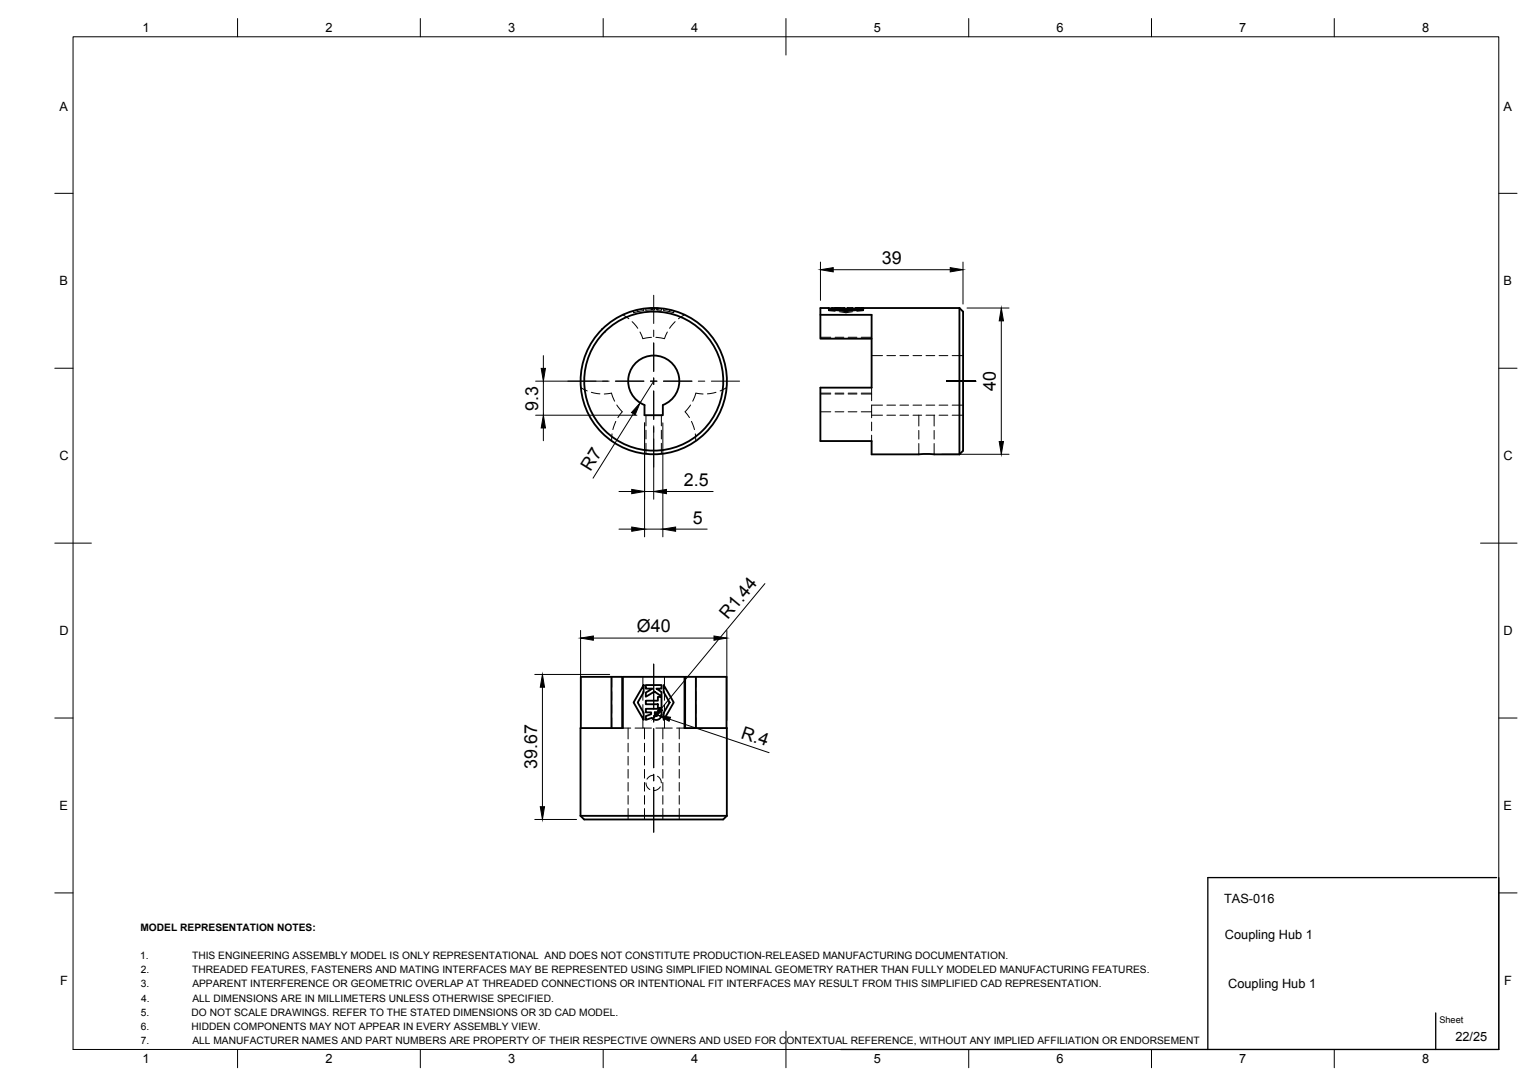
ISO-10303-21;
HEADER;
/* Generated by software containing ST-Developer
 * from STEP Tools, Inc. (www.steptools.com) 
 */

FILE_DESCRIPTION(
/* description */ ('STEP AP214'),
/* implementation_level */ '2;1');

FILE_NAME(
/* name */ 'Coupling Hub 1.step',
/* time_stamp */ '2026-11-15T14:55:55-08:00',
/* author */ (''),
/* organization */ (''),
/* preprocessor_version */ 'ST-DEVELOPER v20.2',
/* originating_system */ 'Autodesk Translation Framework v15.17.0.0',
/* authorisation */ '');

FILE_SCHEMA (('AUTOMOTIVE_DESIGN { 1 0 10303 214 3 1 1 }'));
ENDSEC;

DATA;
#10=MECHANICAL_DESIGN_GEOMETRIC_PRESENTATION_REPRESENTATION('',(#941),#57079);
#66=ELLIPSE('',#25719,40.0000000130718,20.0000000134373);
#67=ELLIPSE('',#25720,39.9999999264935,19.999999930827);
#68=ELLIPSE('',#25721,39.9999999974836,19.9999999977429);
#69=ELLIPSE('',#25722,40.0000000047116,20.0000000045204);
#70=ELLIPSE('',#25723,23.3867968076182,20.);
#71=ELLIPSE('',#25724,23.386796807644,20.);
#72=ELLIPSE('',#25728,24.1243589702644,20.);
#73=ELLIPSE('',#25729,24.124358970134,20.);
#74=ELLIPSE('',#25730,39.999999976902,19.9999999789991);
#75=ELLIPSE('',#25731,40.0000000049323,20.0000000047275);
#76=ELLIPSE('',#25732,39.9999999975502,19.999999997805);
#77=ELLIPSE('',#25733,39.9999999389236,19.9999999427079);
#78=ELLIPSE('',#25748,22.8021268874529,19.5);
#79=ELLIPSE('',#25751,22.8021268874277,19.5);
#80=ELLIPSE('',#25754,23.5212499960078,19.5);
#81=ELLIPSE('',#25764,23.5212499958807,19.5);
#82=ELLIPSE('',#25767,39.0000000024375,19.500000002367);
#83=ELLIPSE('',#25768,39.0000000667235,19.500000064201);
#84=ELLIPSE('',#25769,38.9999999995571,19.5000000004649);
#85=ELLIPSE('',#25770,38.999999996593,19.4999999968888);
#86=ELLIPSE('',#25779,38.9999999955418,19.4999999959037);
#87=ELLIPSE('',#25781,38.999999997527,19.4999999977637);
#88=ELLIPSE('',#25784,39.0000000253793,19.5000000249782);
#89=ELLIPSE('',#25786,39.0000000418424,19.5000000405918);
#844=B_SPLINE_CURVE_WITH_KNOTS('',3,(#51735,#51736,#51737,#51738,#51739,
#51740,#51741,#51742,#51743,#51744,#51745,#51746,#51747,#51748,#51749,#51750,
#51751,#51752),.UNSPECIFIED.,.F.,.F.,(4,2,2,2,2,2,2,2,4),(0.,0.0151925643701926,
0.0303851287403852,0.045584296496648,0.0607834642529108,0.0759910091953897,
0.0911985541378687,0.106391953286869,0.121585352435869),.UNSPECIFIED.);
#845=B_SPLINE_CURVE_WITH_KNOTS('',3,(#51844,#51845,#51846,#51847,#51848,
#51849,#51850,#51851,#51852,#51853,#51854,#51855,#51856,#51857,#51858,#51859,
#51860,#51861),.UNSPECIFIED.,.F.,.F.,(4,2,2,2,2,2,2,2,4),(0.316667444606564,
0.395834141831916,0.475000839057267,0.554167864135198,0.633334889213128,
0.712501914291059,0.791668939368989,0.870835636594341,0.950002333819692),
 .UNSPECIFIED.);
#846=B_SPLINE_CURVE_WITH_KNOTS('',3,(#51863,#51864,#51865,#51866,#51867,
#51868,#51869,#51870,#51871,#51872),.UNSPECIFIED.,.F.,.F.,(4,2,2,2,4),(-1.26666977842626,
-1.18750275334833,-1.10833572827039,-1.02916903104504,-0.950002333819692),
 .UNSPECIFIED.);
#847=B_SPLINE_CURVE_WITH_KNOTS('',3,(#51873,#51874,#51875,#51876,#51877,
#51878,#51879,#51880,#51881,#51882),.UNSPECIFIED.,.F.,.F.,(4,2,2,2,4),(0.950002333819692,
1.02916903104504,1.1083357282704,1.18750275334833,1.26666977842626),
 .UNSPECIFIED.);
#848=B_SPLINE_CURVE_WITH_KNOTS('',3,(#51888,#51889,#51890,#51891,#51892,
#51893,#51894,#51895,#51896,#51897,#51898,#51899,#51900,#51901,#51902,#51903),
 .UNSPECIFIED.,.F.,.F.,(4,2,2,2,2,2,2,4),(-0.779979052988675,-0.757912790448093,
-0.703814302563526,-0.64971581467896,-0.595510917659987,-0.541306020641014,
-0.487185868025911,-0.433065715410808),.UNSPECIFIED.);
#849=B_SPLINE_CURVE_WITH_KNOTS('',3,(#52126,#52127,#52128,#52129,#52130,
#52131,#52132,#52133,#52134,#52135,#52136,#52137,#52138,#52139,#52140,#52141),
 .UNSPECIFIED.,.F.,.F.,(4,2,2,2,2,2,2,4),(0.43308109743951,0.487202501340474,
0.541323905241438,0.595534461493003,0.649745017744569,0.703843614398011,
0.757942211051454,0.780009479202147),.UNSPECIFIED.);
#850=B_SPLINE_CURVE_WITH_KNOTS('',3,(#52173,#52174,#52175,#52176,#52177,
#52178,#52179,#52180,#52181,#52182,#52183,#52184,#52185,#52186,#52187,#52188,
#52189,#52190),.UNSPECIFIED.,.F.,.F.,(4,2,2,2,2,2,2,2,4),(0.121587491028333,
0.136780909575281,0.151974328122229,0.167182628159423,0.182390928196617,
0.197590414964019,0.212789901731421,0.227982441894043,0.243174982056666),
 .UNSPECIFIED.);
#881=SHAPE_REPRESENTATION_RELATIONSHIP('SRR','None',#57269,#910);
#910=ADVANCED_BREP_SHAPE_REPRESENTATION('',(#978),#57061);
#941=STYLED_ITEM('',(#57444),#978);
#978=MANIFOLD_SOLID_BREP('Body1',#24541);
#1139=FACE_BOUND('',#4148,.T.);
#1140=FACE_BOUND('',#4160,.T.);
#1141=FACE_BOUND('',#4166,.T.);
#1142=FACE_BOUND('',#4171,.T.);
#1143=FACE_BOUND('',#4172,.T.);
#1144=FACE_BOUND('',#4173,.T.);
#1145=FACE_BOUND('',#4174,.T.);
#1146=FACE_BOUND('',#4175,.T.);
#1147=FACE_BOUND('',#4225,.T.);
#1550=PLANE('',#25658);
#1551=PLANE('',#25663);
#1552=PLANE('',#25670);
#1553=PLANE('',#25675);
#1554=PLANE('',#25692);
#1555=PLANE('',#25705);
#1556=PLANE('',#25707);
#1557=PLANE('',#25708);
#1558=PLANE('',#25739);
#1559=PLANE('',#25740);
#1560=PLANE('',#25741);
#1561=PLANE('',#25742);
#1562=PLANE('',#25743);
#1563=PLANE('',#25744);
#1564=PLANE('',#25745);
#1565=PLANE('',#25746);
#1566=PLANE('',#25747);
#1567=PLANE('',#25749);
#1568=PLANE('',#25750);
#1569=PLANE('',#25752);
#1570=PLANE('',#25753);
#1571=PLANE('',#25755);
#1572=PLANE('',#25757);
#1573=PLANE('',#25758);
#1574=PLANE('',#25760);
#1575=PLANE('',#25761);
#1576=PLANE('',#25763);
#1577=PLANE('',#25771);
#1578=PLANE('',#25772);
#1579=PLANE('',#25773);
#1580=PLANE('',#25774);
#1581=PLANE('',#25775);
#1582=PLANE('',#25776);
#1583=PLANE('',#25777);
#1584=PLANE('',#25778);
#1585=PLANE('',#25780);
#1586=PLANE('',#25782);
#1587=PLANE('',#25783);
#1588=PLANE('',#25785);
#1589=PLANE('',#25788);
#1590=PLANE('',#25790);
#1591=PLANE('',#25791);
#1592=PLANE('',#25794);
#1593=PLANE('',#25795);
#1594=PLANE('',#25797);
#1595=PLANE('',#25798);
#1596=PLANE('',#25800);
#1597=PLANE('',#25801);
#1598=PLANE('',#25803);
#1599=PLANE('',#25805);
#2122=CONICAL_SURFACE('',#25666,19.5,0.785398163397448);
#2632=FACE_OUTER_BOUND('',#4146,.T.);
#2633=FACE_OUTER_BOUND('',#4147,.T.);
#2634=FACE_OUTER_BOUND('',#4149,.T.);
#2635=FACE_OUTER_BOUND('',#4150,.T.);
#2636=FACE_OUTER_BOUND('',#4151,.T.);
#2637=FACE_OUTER_BOUND('',#4152,.T.);
#2638=FACE_OUTER_BOUND('',#4153,.T.);
#2639=FACE_OUTER_BOUND('',#4154,.T.);
#2640=FACE_OUTER_BOUND('',#4155,.T.);
#2641=FACE_OUTER_BOUND('',#4156,.T.);
#2642=FACE_OUTER_BOUND('',#4157,.T.);
#2643=FACE_OUTER_BOUND('',#4158,.T.);
#2644=FACE_OUTER_BOUND('',#4159,.T.);
#2645=FACE_OUTER_BOUND('',#4161,.T.);
#2646=FACE_OUTER_BOUND('',#4162,.T.);
#2647=FACE_OUTER_BOUND('',#4163,.T.);
#2648=FACE_OUTER_BOUND('',#4164,.T.);
#2649=FACE_OUTER_BOUND('',#4165,.T.);
#2650=FACE_OUTER_BOUND('',#4167,.T.);
#2651=FACE_OUTER_BOUND('',#4168,.T.);
#2652=FACE_OUTER_BOUND('',#4169,.T.);
#2653=FACE_OUTER_BOUND('',#4170,.T.);
#2654=FACE_OUTER_BOUND('',#4176,.T.);
#2655=FACE_OUTER_BOUND('',#4177,.T.);
#2656=FACE_OUTER_BOUND('',#4178,.T.);
#2657=FACE_OUTER_BOUND('',#4179,.T.);
#2658=FACE_OUTER_BOUND('',#4180,.T.);
#2659=FACE_OUTER_BOUND('',#4181,.T.);
#2660=FACE_OUTER_BOUND('',#4182,.T.);
#2661=FACE_OUTER_BOUND('',#4183,.T.);
#2662=FACE_OUTER_BOUND('',#4184,.T.);
#2663=FACE_OUTER_BOUND('',#4185,.T.);
#2664=FACE_OUTER_BOUND('',#4186,.T.);
#2665=FACE_OUTER_BOUND('',#4187,.T.);
#2666=FACE_OUTER_BOUND('',#4188,.T.);
#2667=FACE_OUTER_BOUND('',#4189,.T.);
#2668=FACE_OUTER_BOUND('',#4190,.T.);
#2669=FACE_OUTER_BOUND('',#4191,.T.);
#2670=FACE_OUTER_BOUND('',#4192,.T.);
#2671=FACE_OUTER_BOUND('',#4193,.T.);
#2672=FACE_OUTER_BOUND('',#4194,.T.);
#2673=FACE_OUTER_BOUND('',#4195,.T.);
#2674=FACE_OUTER_BOUND('',#4196,.T.);
#2675=FACE_OUTER_BOUND('',#4197,.T.);
#2676=FACE_OUTER_BOUND('',#4198,.T.);
#2677=FACE_OUTER_BOUND('',#4199,.T.);
#2678=FACE_OUTER_BOUND('',#4200,.T.);
#2679=FACE_OUTER_BOUND('',#4201,.T.);
#2680=FACE_OUTER_BOUND('',#4202,.T.);
#2681=FACE_OUTER_BOUND('',#4203,.T.);
#2682=FACE_OUTER_BOUND('',#4204,.T.);
#2683=FACE_OUTER_BOUND('',#4205,.T.);
#2684=FACE_OUTER_BOUND('',#4206,.T.);
#2685=FACE_OUTER_BOUND('',#4207,.T.);
#2686=FACE_OUTER_BOUND('',#4208,.T.);
#2687=FACE_OUTER_BOUND('',#4209,.T.);
#2688=FACE_OUTER_BOUND('',#4210,.T.);
#2689=FACE_OUTER_BOUND('',#4211,.T.);
#2690=FACE_OUTER_BOUND('',#4212,.T.);
#2691=FACE_OUTER_BOUND('',#4213,.T.);
#2692=FACE_OUTER_BOUND('',#4214,.T.);
#2693=FACE_OUTER_BOUND('',#4215,.T.);
#2694=FACE_OUTER_BOUND('',#4216,.T.);
#2695=FACE_OUTER_BOUND('',#4217,.T.);
#2696=FACE_OUTER_BOUND('',#4218,.T.);
#2697=FACE_OUTER_BOUND('',#4219,.T.);
#2698=FACE_OUTER_BOUND('',#4220,.T.);
#2699=FACE_OUTER_BOUND('',#4221,.T.);
#2700=FACE_OUTER_BOUND('',#4222,.T.);
#2701=FACE_OUTER_BOUND('',#4223,.T.);
#2702=FACE_OUTER_BOUND('',#4224,.T.);
#4146=EDGE_LOOP('',(#18044,#18045,#18046,#18047));
#4147=EDGE_LOOP('',(#18048));
#4148=EDGE_LOOP('',(#18049,#18050,#18051,#18052));
#4149=EDGE_LOOP('',(#18053,#18054,#18055,#18056));
#4150=EDGE_LOOP('',(#18057,#18058,#18059,#18060));
#4151=EDGE_LOOP('',(#18061,#18062,#18063,#18064));
#4152=EDGE_LOOP('',(#18065,#18066,#18067,#18068));
#4153=EDGE_LOOP('',(#18069,#18070,#18071,#18072));
#4154=EDGE_LOOP('',(#18073,#18074,#18075,#18076));
#4155=EDGE_LOOP('',(#18077,#18078,#18079,#18080));
#4156=EDGE_LOOP('',(#18081,#18082,#18083,#18084));
#4157=EDGE_LOOP('',(#18085,#18086,#18087,#18088));
#4158=EDGE_LOOP('',(#18089,#18090,#18091,#18092));
#4159=EDGE_LOOP('',(#18093,#18094,#18095,#18096,#18097,#18098,#18099,#18100,
#18101,#18102,#18103,#18104,#18105));
#4160=EDGE_LOOP('',(#18106,#18107,#18108,#18109));
#4161=EDGE_LOOP('',(#18110,#18111,#18112,#18113));
#4162=EDGE_LOOP('',(#18114,#18115,#18116,#18117));
#4163=EDGE_LOOP('',(#18118,#18119,#18120,#18121));
#4164=EDGE_LOOP('',(#18122,#18123,#18124,#18125));
#4165=EDGE_LOOP('',(#18126,#18127,#18128,#18129));
#4166=EDGE_LOOP('',(#18130));
#4167=EDGE_LOOP('',(#18131,#18132,#18133,#18134));
#4168=EDGE_LOOP('',(#18135,#18136,#18137,#18138));
#4169=EDGE_LOOP('',(#18139,#18140,#18141,#18142,#18143,#18144));
#4170=EDGE_LOOP('',(#18145,#18146,#18147,#18148,#18149,#18150,#18151,#18152,
#18153,#18154,#18155,#18156,#18157,#18158,#18159,#18160,#18161,#18162,#18163,
#18164,#18165));
#4171=EDGE_LOOP('',(#18166,#18167,#18168,#18169,#18170,#18171,#18172,#18173,
#18174));
#4172=EDGE_LOOP('',(#18175,#18176,#18177,#18178,#18179,#18180,#18181,#18182));
#4173=EDGE_LOOP('',(#18183,#18184,#18185,#18186,#18187,#18188));
#4174=EDGE_LOOP('',(#18189,#18190,#18191,#18192,#18193,#18194,#18195,#18196,
#18197,#18198,#18199));
#4175=EDGE_LOOP('',(#18200,#18201,#18202,#18203,#18204,#18205));
#4176=EDGE_LOOP('',(#18206,#18207,#18208,#18209,#18210,#18211,#18212,#18213));
#4177=EDGE_LOOP('',(#18214,#18215,#18216,#18217));
#4178=EDGE_LOOP('',(#18218,#18219,#18220,#18221));
#4179=EDGE_LOOP('',(#18222,#18223,#18224,#18225));
#4180=EDGE_LOOP('',(#18226,#18227,#18228,#18229));
#4181=EDGE_LOOP('',(#18230,#18231,#18232,#18233));
#4182=EDGE_LOOP('',(#18234,#18235,#18236,#18237));
#4183=EDGE_LOOP('',(#18238,#18239,#18240,#18241));
#4184=EDGE_LOOP('',(#18242,#18243,#18244,#18245));
#4185=EDGE_LOOP('',(#18246,#18247,#18248,#18249));
#4186=EDGE_LOOP('',(#18250,#18251,#18252,#18253));
#4187=EDGE_LOOP('',(#18254,#18255,#18256,#18257));
#4188=EDGE_LOOP('',(#18258,#18259,#18260,#18261));
#4189=EDGE_LOOP('',(#18262,#18263,#18264,#18265));
#4190=EDGE_LOOP('',(#18266,#18267,#18268,#18269));
#4191=EDGE_LOOP('',(#18270,#18271,#18272,#18273));
#4192=EDGE_LOOP('',(#18274,#18275,#18276,#18277));
#4193=EDGE_LOOP('',(#18278,#18279,#18280,#18281));
#4194=EDGE_LOOP('',(#18282,#18283,#18284,#18285));
#4195=EDGE_LOOP('',(#18286,#18287,#18288,#18289));
#4196=EDGE_LOOP('',(#18290,#18291,#18292,#18293,#18294,#18295,#18296,#18297,
#18298,#18299,#18300));
#4197=EDGE_LOOP('',(#18301,#18302,#18303,#18304,#18305,#18306));
#4198=EDGE_LOOP('',(#18307,#18308,#18309,#18310));
#4199=EDGE_LOOP('',(#18311,#18312,#18313,#18314));
#4200=EDGE_LOOP('',(#18315,#18316,#18317,#18318));
#4201=EDGE_LOOP('',(#18319,#18320,#18321,#18322));
#4202=EDGE_LOOP('',(#18323,#18324,#18325,#18326));
#4203=EDGE_LOOP('',(#18327,#18328,#18329,#18330));
#4204=EDGE_LOOP('',(#18331,#18332,#18333,#18334));
#4205=EDGE_LOOP('',(#18335,#18336,#18337,#18338));
#4206=EDGE_LOOP('',(#18339,#18340,#18341,#18342));
#4207=EDGE_LOOP('',(#18343,#18344,#18345,#18346));
#4208=EDGE_LOOP('',(#18347,#18348,#18349,#18350));
#4209=EDGE_LOOP('',(#18351,#18352,#18353,#18354));
#4210=EDGE_LOOP('',(#18355,#18356,#18357,#18358,#18359,#18360));
#4211=EDGE_LOOP('',(#18361,#18362,#18363,#18364));
#4212=EDGE_LOOP('',(#18365,#18366,#18367,#18368));
#4213=EDGE_LOOP('',(#18369,#18370,#18371,#18372));
#4214=EDGE_LOOP('',(#18373,#18374,#18375,#18376));
#4215=EDGE_LOOP('',(#18377,#18378,#18379,#18380));
#4216=EDGE_LOOP('',(#18381,#18382,#18383,#18384));
#4217=EDGE_LOOP('',(#18385,#18386,#18387,#18388));
#4218=EDGE_LOOP('',(#18389,#18390,#18391,#18392));
#4219=EDGE_LOOP('',(#18393,#18394,#18395,#18396));
#4220=EDGE_LOOP('',(#18397,#18398,#18399,#18400));
#4221=EDGE_LOOP('',(#18401,#18402,#18403,#18404));
#4222=EDGE_LOOP('',(#18405,#18406,#18407,#18408));
#4223=EDGE_LOOP('',(#18409,#18410,#18411,#18412));
#4224=EDGE_LOOP('',(#18413,#18414,#18415,#18416,#18417,#18418,#18419,#18420,
#18421));
#4225=EDGE_LOOP('',(#18422,#18423,#18424,#18425));
#5739=LINE('',#51720,#7706);
#5740=LINE('',#51724,#7707);
#5741=LINE('',#51725,#7708);
#5742=LINE('',#51729,#7709);
#5743=LINE('',#51733,#7710);
#5744=LINE('',#51754,#7711);
#5745=LINE('',#51778,#7712);
#5746=LINE('',#51779,#7713);
#5747=LINE('',#51782,#7714);
#5748=LINE('',#51785,#7715);
#5749=LINE('',#51788,#7716);
#5750=LINE('',#51791,#7717);
#5751=LINE('',#51794,#7718);
#5752=LINE('',#51798,#7719);
#5753=LINE('',#51803,#7720);
#5754=LINE('',#51818,#7721);
#5755=LINE('',#51820,#7722);
#5756=LINE('',#51822,#7723);
#5757=LINE('',#51825,#7724);
#5758=LINE('',#51827,#7725);
#5759=LINE('',#51829,#7726);
#5760=LINE('',#51831,#7727);
#5761=LINE('',#51832,#7728);
#5762=LINE('',#51834,#7729);
#5763=LINE('',#51835,#7730);
#5764=LINE('',#51842,#7731);
#5765=LINE('',#51884,#7732);
#5766=LINE('',#51885,#7733);
#5767=LINE('',#51907,#7734);
#5768=LINE('',#51911,#7735);
#5769=LINE('',#51915,#7736);
#5770=LINE('',#51918,#7737);
#5771=LINE('',#51923,#7738);
#5772=LINE('',#51927,#7739);
#5773=LINE('',#51931,#7740);
#5774=LINE('',#51934,#7741);
#5775=LINE('',#51937,#7742);
#5776=LINE('',#51943,#7743);
#5777=LINE('',#51951,#7744);
#5778=LINE('',#51957,#7745);
#5779=LINE('',#51961,#7746);
#5780=LINE('',#51967,#7747);
#5781=LINE('',#51973,#7748);
#5782=LINE('',#51979,#7749);
#5783=LINE('',#51986,#7750);
#5784=LINE('',#51990,#7751);
#5785=LINE('',#51994,#7752);
#5786=LINE('',#51997,#7753);
#5787=LINE('',#51999,#7754);
#5788=LINE('',#52000,#7755);
#5789=LINE('',#52002,#7756);
#5790=LINE('',#52004,#7757);
#5791=LINE('',#52006,#7758);
#5792=LINE('',#52008,#7759);
#5793=LINE('',#52010,#7760);
#5794=LINE('',#52012,#7761);
#5795=LINE('',#52016,#7762);
#5796=LINE('',#52019,#7763);
#5797=LINE('',#52022,#7764);
#5798=LINE('',#52023,#7765);
#5799=LINE('',#52026,#7766);
#5800=LINE('',#52030,#7767);
#5801=LINE('',#52032,#7768);
#5802=LINE('',#52033,#7769);
#5803=LINE('',#52036,#7770);
#5804=LINE('',#52040,#7771);
#5805=LINE('',#52044,#7772);
#5806=LINE('',#52045,#7773);
#5807=LINE('',#52048,#7774);
#5808=LINE('',#52052,#7775);
#5809=LINE('',#52053,#7776);
#5810=LINE('',#52064,#7777);
#5811=LINE('',#52070,#7778);
#5812=LINE('',#52073,#7779);
#5813=LINE('',#52074,#7780);
#5814=LINE('',#52076,#7781);
#5815=LINE('',#52078,#7782);
#5816=LINE('',#52080,#7783);
#5817=LINE('',#52082,#7784);
#5818=LINE('',#52086,#7785);
#5819=LINE('',#52088,#7786);
#5820=LINE('',#52089,#7787);
#5821=LINE('',#52092,#7788);
#5822=LINE('',#52096,#7789);
#5823=LINE('',#52100,#7790);
#5824=LINE('',#52101,#7791);
#5825=LINE('',#52105,#7792);
#5826=LINE('',#52111,#7793);
#5827=LINE('',#52114,#7794);
#5828=LINE('',#52117,#7795);
#5829=LINE('',#52118,#7796);
#5830=LINE('',#52121,#7797);
#5831=LINE('',#52125,#7798);
#5832=LINE('',#52144,#7799);
#5833=LINE('',#52145,#7800);
#5834=LINE('',#52148,#7801);
#5835=LINE('',#52151,#7802);
#5836=LINE('',#52154,#7803);
#5837=LINE('',#52155,#7804);
#5838=LINE('',#52158,#7805);
#5839=LINE('',#52162,#7806);
#5840=LINE('',#52163,#7807);
#5841=LINE('',#52166,#7808);
#5842=LINE('',#52169,#7809);
#5843=LINE('',#52172,#7810);
#5844=LINE('',#52192,#7811);
#7706=VECTOR('',#29529,1000.);
#7707=VECTOR('',#29532,1000.);
#7708=VECTOR('',#29533,1000.);
#7709=VECTOR('',#29538,19.5);
#7710=VECTOR('',#29541,1000.);
#7711=VECTOR('',#29542,1000.);
#7712=VECTOR('',#29569,1000.);
#7713=VECTOR('',#29570,1000.);
#7714=VECTOR('',#29573,1000.);
#7715=VECTOR('',#29576,1000.);
#7716=VECTOR('',#29579,1000.);
#7717=VECTOR('',#29582,1000.);
#7718=VECTOR('',#29585,1000.);
#7719=VECTOR('',#29590,1000.);
#7720=VECTOR('',#29597,1000.);
#7721=VECTOR('',#29614,1000.);
#7722=VECTOR('',#29615,1000.);
#7723=VECTOR('',#29616,1000.);
#7724=VECTOR('',#29621,1000.);
#7725=VECTOR('',#29624,1000.);
#7726=VECTOR('',#29627,1000.);
#7727=VECTOR('',#29630,1000.);
#7728=VECTOR('',#29631,1000.);
#7729=VECTOR('',#29634,1000.);
#7730=VECTOR('',#29635,1000.);
#7731=VECTOR('',#29644,2.1);
#7732=VECTOR('',#29647,20.);
#7733=VECTOR('',#29648,20.);
#7734=VECTOR('',#29651,1000.);
#7735=VECTOR('',#29654,1000.);
#7736=VECTOR('',#29657,1000.);
#7737=VECTOR('',#29660,1000.);
#7738=VECTOR('',#29663,1000.);
#7739=VECTOR('',#29666,1000.);
#7740=VECTOR('',#29669,1000.);
#7741=VECTOR('',#29672,1000.);
#7742=VECTOR('',#29673,1000.);
#7743=VECTOR('',#29678,1000.);
#7744=VECTOR('',#29685,1000.);
#7745=VECTOR('',#29690,1000.);
#7746=VECTOR('',#29693,1000.);
#7747=VECTOR('',#29698,1000.);
#7748=VECTOR('',#29703,1000.);
#7749=VECTOR('',#29708,1000.);
#7750=VECTOR('',#29715,1000.);
#7751=VECTOR('',#29718,1000.);
#7752=VECTOR('',#29721,1000.);
#7753=VECTOR('',#29724,1000.);
#7754=VECTOR('',#29727,1000.);
#7755=VECTOR('',#29728,1000.);
#7756=VECTOR('',#29731,1000.);
#7757=VECTOR('',#29734,1000.);
#7758=VECTOR('',#29737,1000.);
#7759=VECTOR('',#29740,1000.);
#7760=VECTOR('',#29743,1000.);
#7761=VECTOR('',#29746,1000.);
#7762=VECTOR('',#29751,1000.);
#7763=VECTOR('',#29754,1000.);
#7764=VECTOR('',#29757,1000.);
#7765=VECTOR('',#29758,1000.);
#7766=VECTOR('',#29761,1000.);
#7767=VECTOR('',#29766,1000.);
#7768=VECTOR('',#29767,1000.);
#7769=VECTOR('',#29768,1000.);
#7770=VECTOR('',#29771,1000.);
#7771=VECTOR('',#29776,1000.);
#7772=VECTOR('',#29781,1000.);
#7773=VECTOR('',#29782,1000.);
#7774=VECTOR('',#29785,1000.);
#7775=VECTOR('',#29790,1000.);
#7776=VECTOR('',#29791,1000.);
#7777=VECTOR('',#29806,1000.);
#7778=VECTOR('',#29811,1000.);
#7779=VECTOR('',#29816,1000.);
#7780=VECTOR('',#29817,1000.);
#7781=VECTOR('',#29820,1000.);
#7782=VECTOR('',#29823,1000.);
#7783=VECTOR('',#29826,1000.);
#7784=VECTOR('',#29829,1000.);
#7785=VECTOR('',#29834,1000.);
#7786=VECTOR('',#29835,1000.);
#7787=VECTOR('',#29836,1000.);
#7788=VECTOR('',#29839,1000.);
#7789=VECTOR('',#29844,1000.);
#7790=VECTOR('',#29849,1000.);
#7791=VECTOR('',#29850,1000.);
#7792=VECTOR('',#29855,1000.);
#7793=VECTOR('',#29864,1000.);
#7794=VECTOR('',#29867,1000.);
#7795=VECTOR('',#29870,1000.);
#7796=VECTOR('',#29871,1000.);
#7797=VECTOR('',#29874,1000.);
#7798=VECTOR('',#29879,1000.);
#7799=VECTOR('',#29882,1000.);
#7800=VECTOR('',#29883,1000.);
#7801=VECTOR('',#29886,1000.);
#7802=VECTOR('',#29889,1000.);
#7803=VECTOR('',#29892,1000.);
#7804=VECTOR('',#29893,1000.);
#7805=VECTOR('',#29896,1000.);
#7806=VECTOR('',#29901,1000.);
#7807=VECTOR('',#29902,1000.);
#7808=VECTOR('',#29905,1000.);
#7809=VECTOR('',#29910,1000.);
#7810=VECTOR('',#29913,1000.);
#7811=VECTOR('',#29916,1000.);
#9554=CIRCLE('',#25659,11.5);
#9555=CIRCLE('',#25660,20.);
#9556=CIRCLE('',#25661,11.5);
#9557=CIRCLE('',#25662,12.);
#9558=CIRCLE('',#25664,19.);
#9559=CIRCLE('',#25665,7.);
#9560=CIRCLE('',#25667,20.);
#9561=CIRCLE('',#25669,20.);
#9562=CIRCLE('',#25671,11.5);
#9563=CIRCLE('',#25672,20.);
#9564=CIRCLE('',#25673,11.5);
#9565=CIRCLE('',#25674,12.);
#9566=CIRCLE('',#25676,11.5);
#9567=CIRCLE('',#25677,12.);
#9568=CIRCLE('',#25678,11.5);
#9569=CIRCLE('',#25679,20.);
#9570=CIRCLE('',#25681,11.5);
#9571=CIRCLE('',#25683,12.);
#9572=CIRCLE('',#25685,12.);
#9573=CIRCLE('',#25687,12.);
#9574=CIRCLE('',#25689,11.5);
#9575=CIRCLE('',#25691,11.5);
#9576=CIRCLE('',#25693,20.);
#9577=CIRCLE('',#25694,11.5);
#9578=CIRCLE('',#25695,20.);
#9579=CIRCLE('',#25696,20.);
#9580=CIRCLE('',#25697,11.5);
#9581=CIRCLE('',#25698,20.);
#9582=CIRCLE('',#25699,11.5);
#9583=CIRCLE('',#25700,7.);
#9584=CIRCLE('',#25706,2.1);
#9585=CIRCLE('',#25711,22.3311974134124);
#9586=CIRCLE('',#25712,22.32884051476);
#9587=CIRCLE('',#25713,20.);
#9588=CIRCLE('',#25714,20.);
#9589=CIRCLE('',#25715,20.);
#9590=CIRCLE('',#25716,20.);
#9591=CIRCLE('',#25717,20.);
#9592=CIRCLE('',#25718,20.);
#9593=CIRCLE('',#25725,20.);
#9594=CIRCLE('',#25726,20.);
#9595=CIRCLE('',#25727,20.);
#9596=CIRCLE('',#25735,19.5);
#9597=CIRCLE('',#25736,19.5);
#9598=CIRCLE('',#25737,19.5);
#9599=CIRCLE('',#25738,19.5);
#9600=CIRCLE('',#25756,19.5);
#9601=CIRCLE('',#25759,19.5);
#9602=CIRCLE('',#25762,19.5);
#9603=CIRCLE('',#25789,21.7696935948967);
#9604=CIRCLE('',#25792,21.7721107487055);
#9605=CIRCLE('',#25796,19.5);
#9606=CIRCLE('',#25799,19.5);
#9607=CIRCLE('',#25802,19.5);
#10947=VERTEX_POINT('',#51707);
#10948=VERTEX_POINT('',#51708);
#10949=VERTEX_POINT('',#51710);
#10950=VERTEX_POINT('',#51712);
#10951=VERTEX_POINT('',#51716);
#10952=VERTEX_POINT('',#51718);
#10953=VERTEX_POINT('',#51719);
#10954=VERTEX_POINT('',#51721);
#10955=VERTEX_POINT('',#51723);
#10956=VERTEX_POINT('',#51727);
#10957=VERTEX_POINT('',#51731);
#10958=VERTEX_POINT('',#51732);
#10959=VERTEX_POINT('',#51734);
#10960=VERTEX_POINT('',#51753);
#10961=VERTEX_POINT('',#51757);
#10962=VERTEX_POINT('',#51758);
#10963=VERTEX_POINT('',#51760);
#10964=VERTEX_POINT('',#51762);
#10965=VERTEX_POINT('',#51766);
#10966=VERTEX_POINT('',#51767);
#10967=VERTEX_POINT('',#51769);
#10968=VERTEX_POINT('',#51771);
#10969=VERTEX_POINT('',#51775);
#10970=VERTEX_POINT('',#51776);
#10971=VERTEX_POINT('',#51781);
#10972=VERTEX_POINT('',#51783);
#10973=VERTEX_POINT('',#51787);
#10974=VERTEX_POINT('',#51789);
#10975=VERTEX_POINT('',#51793);
#10976=VERTEX_POINT('',#51797);
#10977=VERTEX_POINT('',#51801);
#10978=VERTEX_POINT('',#51805);
#10979=VERTEX_POINT('',#51807);
#10980=VERTEX_POINT('',#51809);
#10981=VERTEX_POINT('',#51811);
#10982=VERTEX_POINT('',#51816);
#10983=VERTEX_POINT('',#51817);
#10984=VERTEX_POINT('',#51819);
#10985=VERTEX_POINT('',#51821);
#10986=VERTEX_POINT('',#51836);
#10987=VERTEX_POINT('',#51841);
#10988=VERTEX_POINT('',#51843);
#10989=VERTEX_POINT('',#51862);
#10990=VERTEX_POINT('',#51886);
#10991=VERTEX_POINT('',#51887);
#10992=VERTEX_POINT('',#51904);
#10993=VERTEX_POINT('',#51906);
#10994=VERTEX_POINT('',#51908);
#10995=VERTEX_POINT('',#51910);
#10996=VERTEX_POINT('',#51912);
#10997=VERTEX_POINT('',#51914);
#10998=VERTEX_POINT('',#51916);
#10999=VERTEX_POINT('',#51919);
#11000=VERTEX_POINT('',#51920);
#11001=VERTEX_POINT('',#51922);
#11002=VERTEX_POINT('',#51924);
#11003=VERTEX_POINT('',#51926);
#11004=VERTEX_POINT('',#51928);
#11005=VERTEX_POINT('',#51930);
#11006=VERTEX_POINT('',#51932);
#11007=VERTEX_POINT('',#51935);
#11008=VERTEX_POINT('',#51936);
#11009=VERTEX_POINT('',#51938);
#11010=VERTEX_POINT('',#51940);
#11011=VERTEX_POINT('',#51942);
#11012=VERTEX_POINT('',#51944);
#11013=VERTEX_POINT('',#51947);
#11014=VERTEX_POINT('',#51948);
#11015=VERTEX_POINT('',#51950);
#11016=VERTEX_POINT('',#51952);
#11017=VERTEX_POINT('',#51954);
#11018=VERTEX_POINT('',#51956);
#11019=VERTEX_POINT('',#51958);
#11020=VERTEX_POINT('',#51960);
#11021=VERTEX_POINT('',#51962);
#11022=VERTEX_POINT('',#51964);
#11023=VERTEX_POINT('',#51966);
#11024=VERTEX_POINT('',#51969);
#11025=VERTEX_POINT('',#51970);
#11026=VERTEX_POINT('',#51972);
#11027=VERTEX_POINT('',#51974);
#11028=VERTEX_POINT('',#51976);
#11029=VERTEX_POINT('',#51978);
#11030=VERTEX_POINT('',#51982);
#11031=VERTEX_POINT('',#51983);
#11032=VERTEX_POINT('',#51985);
#11033=VERTEX_POINT('',#51987);
#11034=VERTEX_POINT('',#51989);
#11035=VERTEX_POINT('',#51991);
#11036=VERTEX_POINT('',#51993);
#11037=VERTEX_POINT('',#51995);
#11038=VERTEX_POINT('',#52015);
#11039=VERTEX_POINT('',#52017);
#11040=VERTEX_POINT('',#52021);
#11041=VERTEX_POINT('',#52025);
#11042=VERTEX_POINT('',#52029);
#11043=VERTEX_POINT('',#52031);
#11044=VERTEX_POINT('',#52035);
#11045=VERTEX_POINT('',#52039);
#11046=VERTEX_POINT('',#52043);
#11047=VERTEX_POINT('',#52047);
#11048=VERTEX_POINT('',#52051);
#11049=VERTEX_POINT('',#52060);
#11050=VERTEX_POINT('',#52061);
#11051=VERTEX_POINT('',#52063);
#11052=VERTEX_POINT('',#52065);
#11053=VERTEX_POINT('',#52067);
#11054=VERTEX_POINT('',#52069);
#11055=VERTEX_POINT('',#52085);
#11056=VERTEX_POINT('',#52087);
#11057=VERTEX_POINT('',#52091);
#11058=VERTEX_POINT('',#52095);
#11059=VERTEX_POINT('',#52099);
#11060=VERTEX_POINT('',#52103);
#11061=VERTEX_POINT('',#52110);
#11062=VERTEX_POINT('',#52112);
#11063=VERTEX_POINT('',#52116);
#11064=VERTEX_POINT('',#52120);
#11065=VERTEX_POINT('',#52124);
#11066=VERTEX_POINT('',#52143);
#11067=VERTEX_POINT('',#52147);
#11068=VERTEX_POINT('',#52149);
#11069=VERTEX_POINT('',#52153);
#11070=VERTEX_POINT('',#52157);
#11071=VERTEX_POINT('',#52161);
#11072=VERTEX_POINT('',#52165);
#11073=VERTEX_POINT('',#52171);
#13567=EDGE_CURVE('',#10947,#10948,#9554,.T.);
#13568=EDGE_CURVE('',#10949,#10948,#9555,.T.);
#13569=EDGE_CURVE('',#10949,#10950,#9556,.T.);
#13570=EDGE_CURVE('',#10950,#10947,#9557,.T.);
#13571=EDGE_CURVE('',#10951,#10951,#9558,.T.);
#13572=EDGE_CURVE('',#10952,#10953,#5739,.T.);
#13573=EDGE_CURVE('',#10953,#10954,#9559,.T.);
#13574=EDGE_CURVE('',#10954,#10955,#5740,.T.);
#13575=EDGE_CURVE('',#10955,#10952,#5741,.T.);
#13576=EDGE_CURVE('',#10956,#10956,#9560,.T.);
#13577=EDGE_CURVE('',#10956,#10951,#5742,.T.);
#13578=EDGE_CURVE('',#10957,#10958,#5743,.T.);
#13579=EDGE_CURVE('',#10958,#10959,#844,.T.);
#13580=EDGE_CURVE('',#10959,#10960,#5744,.T.);
#13581=EDGE_CURVE('',#10960,#10957,#9561,.T.);
#13582=EDGE_CURVE('',#10961,#10962,#9562,.T.);
#13583=EDGE_CURVE('',#10963,#10962,#9563,.T.);
#13584=EDGE_CURVE('',#10963,#10964,#9564,.T.);
#13585=EDGE_CURVE('',#10964,#10961,#9565,.T.);
#13586=EDGE_CURVE('',#10965,#10966,#9566,.T.);
#13587=EDGE_CURVE('',#10966,#10967,#9567,.T.);
#13588=EDGE_CURVE('',#10967,#10968,#9568,.T.);
#13589=EDGE_CURVE('',#10965,#10968,#9569,.T.);
#13590=EDGE_CURVE('',#10969,#10970,#9570,.T.);
#13591=EDGE_CURVE('',#10948,#10970,#5745,.T.);
#13592=EDGE_CURVE('',#10969,#10947,#5746,.T.);
#13593=EDGE_CURVE('',#10966,#10971,#5747,.T.);
#13594=EDGE_CURVE('',#10971,#10972,#9571,.T.);
#13595=EDGE_CURVE('',#10972,#10967,#5748,.T.);
#13596=EDGE_CURVE('',#10964,#10973,#5749,.T.);
#13597=EDGE_CURVE('',#10973,#10974,#9572,.T.);
#13598=EDGE_CURVE('',#10974,#10961,#5750,.T.);
#13599=EDGE_CURVE('',#10950,#10975,#5751,.T.);
#13600=EDGE_CURVE('',#10975,#10969,#9573,.T.);
#13601=EDGE_CURVE('',#10976,#10963,#5752,.T.);
#13602=EDGE_CURVE('',#10976,#10973,#9574,.T.);
#13603=EDGE_CURVE('',#10972,#10977,#9575,.T.);
#13604=EDGE_CURVE('',#10968,#10977,#5753,.T.);
#13605=EDGE_CURVE('',#10970,#10978,#9576,.T.);
#13606=EDGE_CURVE('',#10979,#10975,#9577,.T.);
#13607=EDGE_CURVE('',#10980,#10979,#9578,.T.);
#13608=EDGE_CURVE('',#10981,#10980,#9579,.T.);
#13609=EDGE_CURVE('',#10974,#10981,#9580,.T.);
#13610=EDGE_CURVE('',#10977,#10976,#9581,.T.);
#13611=EDGE_CURVE('',#10978,#10971,#9582,.T.);
#13612=EDGE_CURVE('',#10982,#10983,#5754,.T.);
#13613=EDGE_CURVE('',#10983,#10984,#5755,.T.);
#13614=EDGE_CURVE('',#10984,#10985,#5756,.T.);
#13615=EDGE_CURVE('',#10985,#10982,#9583,.T.);
#13616=EDGE_CURVE('',#10979,#10949,#5757,.T.);
#13617=EDGE_CURVE('',#10962,#10981,#5758,.T.);
#13618=EDGE_CURVE('',#10978,#10965,#5759,.T.);
#13619=EDGE_CURVE('',#10954,#10985,#5760,.T.);
#13620=EDGE_CURVE('',#10982,#10953,#5761,.T.);
#13621=EDGE_CURVE('',#10952,#10983,#5762,.T.);
#13622=EDGE_CURVE('',#10984,#10955,#5763,.T.);
#13623=EDGE_CURVE('',#10986,#10986,#9584,.T.);
#13624=EDGE_CURVE('',#10986,#10987,#5764,.T.);
#13625=EDGE_CURVE('',#10988,#10987,#845,.T.);
#13626=EDGE_CURVE('',#10989,#10988,#846,.T.);
#13627=EDGE_CURVE('',#10987,#10989,#847,.T.);
#13628=EDGE_CURVE('',#10956,#10987,#5765,.T.);
#13629=EDGE_CURVE('',#10988,#10980,#5766,.T.);
#13630=EDGE_CURVE('',#10990,#10991,#848,.F.);
#13631=EDGE_CURVE('',#10991,#10992,#9585,.T.);
#13632=EDGE_CURVE('',#10992,#10993,#5767,.T.);
#13633=EDGE_CURVE('',#10993,#10994,#9586,.T.);
#13634=EDGE_CURVE('',#10994,#10995,#5768,.T.);
#13635=EDGE_CURVE('',#10995,#10996,#9587,.T.);
#13636=EDGE_CURVE('',#10996,#10997,#5769,.T.);
#13637=EDGE_CURVE('',#10997,#10998,#9588,.T.);
#13638=EDGE_CURVE('',#10998,#10990,#5770,.T.);
#13639=EDGE_CURVE('',#10999,#11000,#9589,.T.);
#13640=EDGE_CURVE('',#11000,#11001,#5771,.T.);
#13641=EDGE_CURVE('',#11001,#11002,#9590,.T.);
#13642=EDGE_CURVE('',#11002,#11003,#5772,.T.);
#13643=EDGE_CURVE('',#11003,#11004,#9591,.T.);
#13644=EDGE_CURVE('',#11004,#11005,#5773,.T.);
#13645=EDGE_CURVE('',#11005,#11006,#9592,.T.);
#13646=EDGE_CURVE('',#11006,#10999,#5774,.T.);
#13647=EDGE_CURVE('',#11007,#11008,#5775,.T.);
#13648=EDGE_CURVE('',#11008,#11009,#66,.T.);
#13649=EDGE_CURVE('',#11009,#11010,#67,.T.);
#13650=EDGE_CURVE('',#11010,#11011,#5776,.T.);
#13651=EDGE_CURVE('',#11011,#11012,#68,.T.);
#13652=EDGE_CURVE('',#11012,#11007,#69,.T.);
#13653=EDGE_CURVE('',#11013,#11014,#70,.F.);
#13654=EDGE_CURVE('',#11014,#11015,#5777,.T.);
#13655=EDGE_CURVE('',#11015,#11016,#71,.T.);
#13656=EDGE_CURVE('',#11016,#11017,#9593,.T.);
#13657=EDGE_CURVE('',#11017,#11018,#5778,.T.);
#13658=EDGE_CURVE('',#11018,#11019,#9594,.T.);
#13659=EDGE_CURVE('',#11019,#11020,#5779,.T.);
#13660=EDGE_CURVE('',#11020,#11021,#9595,.T.);
#13661=EDGE_CURVE('',#11021,#11022,#72,.T.);
#13662=EDGE_CURVE('',#11022,#11023,#5780,.T.);
#13663=EDGE_CURVE('',#11023,#11013,#73,.T.);
#13664=EDGE_CURVE('',#11024,#11025,#74,.T.);
#13665=EDGE_CURVE('',#11025,#11026,#5781,.T.);
#13666=EDGE_CURVE('',#11026,#11027,#75,.T.);
#13667=EDGE_CURVE('',#11027,#11028,#76,.T.);
#13668=EDGE_CURVE('',#11028,#11029,#5782,.T.);
#13669=EDGE_CURVE('',#11029,#11024,#77,.T.);
#13670=EDGE_CURVE('',#11030,#11031,#9596,.T.);
#13671=EDGE_CURVE('',#11031,#11032,#5783,.T.);
#13672=EDGE_CURVE('',#11032,#11033,#9597,.T.);
#13673=EDGE_CURVE('',#11033,#11034,#5784,.T.);
#13674=EDGE_CURVE('',#11034,#11035,#9598,.T.);
#13675=EDGE_CURVE('',#11035,#11036,#5785,.T.);
#13676=EDGE_CURVE('',#11036,#11037,#9599,.T.);
#13677=EDGE_CURVE('',#11037,#11030,#5786,.T.);
#13678=EDGE_CURVE('',#11037,#11001,#5787,.T.);
#13679=EDGE_CURVE('',#11036,#11002,#5788,.T.);
#13680=EDGE_CURVE('',#11030,#11000,#5789,.T.);
#13681=EDGE_CURVE('',#11035,#11003,#5790,.T.);
#13682=EDGE_CURVE('',#11034,#11004,#5791,.T.);
#13683=EDGE_CURVE('',#11033,#11005,#5792,.T.);
#13684=EDGE_CURVE('',#11032,#11006,#5793,.T.);
#13685=EDGE_CURVE('',#11031,#10999,#5794,.T.);
#13686=EDGE_CURVE('',#11038,#11015,#5795,.T.);
#13687=EDGE_CURVE('',#11039,#11038,#78,.T.);
#13688=EDGE_CURVE('',#11039,#11016,#5796,.T.);
#13689=EDGE_CURVE('',#11040,#11014,#5797,.T.);
#13690=EDGE_CURVE('',#11038,#11040,#5798,.T.);
#13691=EDGE_CURVE('',#11041,#11013,#5799,.T.);
#13692=EDGE_CURVE('',#11040,#11041,#79,.F.);
#13693=EDGE_CURVE('',#11042,#11022,#5800,.T.);
#13694=EDGE_CURVE('',#11043,#11042,#5801,.T.);
#13695=EDGE_CURVE('',#11043,#11023,#5802,.T.);
#13696=EDGE_CURVE('',#11044,#11021,#5803,.T.);
#13697=EDGE_CURVE('',#11042,#11044,#80,.T.);
#13698=EDGE_CURVE('',#11045,#11020,#5804,.T.);
#13699=EDGE_CURVE('',#11044,#11045,#9600,.T.);
#13700=EDGE_CURVE('',#11046,#11019,#5805,.T.);
#13701=EDGE_CURVE('',#11045,#11046,#5806,.T.);
#13702=EDGE_CURVE('',#11047,#11018,#5807,.T.);
#13703=EDGE_CURVE('',#11046,#11047,#9601,.T.);
#13704=EDGE_CURVE('',#11048,#11017,#5808,.T.);
#13705=EDGE_CURVE('',#11047,#11048,#5809,.T.);
#13706=EDGE_CURVE('',#11048,#11039,#9602,.T.);
#13707=EDGE_CURVE('',#11041,#11043,#81,.T.);
#13708=EDGE_CURVE('',#11049,#11050,#82,.T.);
#13709=EDGE_CURVE('',#11050,#11051,#5810,.T.);
#13710=EDGE_CURVE('',#11051,#11052,#83,.T.);
#13711=EDGE_CURVE('',#11052,#11053,#84,.T.);
#13712=EDGE_CURVE('',#11053,#11054,#5811,.T.);
#13713=EDGE_CURVE('',#11054,#11049,#85,.T.);
#13714=EDGE_CURVE('',#11052,#11009,#5812,.T.);
#13715=EDGE_CURVE('',#11051,#11010,#5813,.T.);
#13716=EDGE_CURVE('',#11053,#11008,#5814,.T.);
#13717=EDGE_CURVE('',#11050,#11011,#5815,.T.);
#13718=EDGE_CURVE('',#11049,#11012,#5816,.T.);
#13719=EDGE_CURVE('',#11054,#11007,#5817,.T.);
#13720=EDGE_CURVE('',#11055,#11028,#5818,.T.);
#13721=EDGE_CURVE('',#11056,#11055,#5819,.T.);
#13722=EDGE_CURVE('',#11056,#11029,#5820,.T.);
#13723=EDGE_CURVE('',#11057,#11027,#5821,.T.);
#13724=EDGE_CURVE('',#11055,#11057,#86,.T.);
#13725=EDGE_CURVE('',#11058,#11026,#5822,.T.);
#13726=EDGE_CURVE('',#11057,#11058,#87,.T.);
#13727=EDGE_CURVE('',#11059,#11025,#5823,.T.);
#13728=EDGE_CURVE('',#11058,#11059,#5824,.T.);
#13729=EDGE_CURVE('',#11060,#11056,#88,.T.);
#13730=EDGE_CURVE('',#11060,#11024,#5825,.T.);
#13731=EDGE_CURVE('',#11059,#11060,#89,.T.);
#13732=EDGE_CURVE('',#11061,#10993,#5826,.T.);
#13733=EDGE_CURVE('',#11062,#11061,#9603,.T.);
#13734=EDGE_CURVE('',#11062,#10994,#5827,.T.);
#13735=EDGE_CURVE('',#11063,#10992,#5828,.T.);
#13736=EDGE_CURVE('',#11061,#11063,#5829,.T.);
#13737=EDGE_CURVE('',#11064,#10991,#5830,.T.);
#13738=EDGE_CURVE('',#11063,#11064,#9604,.T.);
#13739=EDGE_CURVE('',#11065,#10990,#5831,.T.);
#13740=EDGE_CURVE('',#11064,#11065,#849,.F.);
#13741=EDGE_CURVE('',#11066,#10998,#5832,.T.);
#13742=EDGE_CURVE('',#11065,#11066,#5833,.T.);
#13743=EDGE_CURVE('',#11067,#10960,#5834,.T.);
#13744=EDGE_CURVE('',#11068,#11067,#9605,.T.);
#13745=EDGE_CURVE('',#11068,#10957,#5835,.T.);
#13746=EDGE_CURVE('',#11069,#10959,#5836,.T.);
#13747=EDGE_CURVE('',#11067,#11069,#5837,.T.);
#13748=EDGE_CURVE('',#11070,#10997,#5838,.T.);
#13749=EDGE_CURVE('',#11066,#11070,#9606,.T.);
#13750=EDGE_CURVE('',#11071,#10996,#5839,.T.);
#13751=EDGE_CURVE('',#11070,#11071,#5840,.T.);
#13752=EDGE_CURVE('',#11072,#10995,#5841,.T.);
#13753=EDGE_CURVE('',#11071,#11072,#9607,.T.);
#13754=EDGE_CURVE('',#11072,#11062,#5842,.T.);
#13755=EDGE_CURVE('',#11073,#10958,#5843,.T.);
#13756=EDGE_CURVE('',#11069,#11073,#850,.T.);
#13757=EDGE_CURVE('',#11073,#11068,#5844,.T.);
#18044=ORIENTED_EDGE('',*,*,#13567,.T.);
#18045=ORIENTED_EDGE('',*,*,#13568,.F.);
#18046=ORIENTED_EDGE('',*,*,#13569,.T.);
#18047=ORIENTED_EDGE('',*,*,#13570,.T.);
#18048=ORIENTED_EDGE('',*,*,#13571,.T.);
#18049=ORIENTED_EDGE('',*,*,#13572,.T.);
#18050=ORIENTED_EDGE('',*,*,#13573,.T.);
#18051=ORIENTED_EDGE('',*,*,#13574,.T.);
#18052=ORIENTED_EDGE('',*,*,#13575,.T.);
#18053=ORIENTED_EDGE('',*,*,#13576,.T.);
#18054=ORIENTED_EDGE('',*,*,#13577,.T.);
#18055=ORIENTED_EDGE('',*,*,#13571,.F.);
#18056=ORIENTED_EDGE('',*,*,#13577,.F.);
#18057=ORIENTED_EDGE('',*,*,#13578,.T.);
#18058=ORIENTED_EDGE('',*,*,#13579,.T.);
#18059=ORIENTED_EDGE('',*,*,#13580,.T.);
#18060=ORIENTED_EDGE('',*,*,#13581,.T.);
#18061=ORIENTED_EDGE('',*,*,#13582,.T.);
#18062=ORIENTED_EDGE('',*,*,#13583,.F.);
#18063=ORIENTED_EDGE('',*,*,#13584,.T.);
#18064=ORIENTED_EDGE('',*,*,#13585,.T.);
#18065=ORIENTED_EDGE('',*,*,#13586,.T.);
#18066=ORIENTED_EDGE('',*,*,#13587,.T.);
#18067=ORIENTED_EDGE('',*,*,#13588,.T.);
#18068=ORIENTED_EDGE('',*,*,#13589,.F.);
#18069=ORIENTED_EDGE('',*,*,#13590,.T.);
#18070=ORIENTED_EDGE('',*,*,#13591,.F.);
#18071=ORIENTED_EDGE('',*,*,#13567,.F.);
#18072=ORIENTED_EDGE('',*,*,#13592,.F.);
#18073=ORIENTED_EDGE('',*,*,#13587,.F.);
#18074=ORIENTED_EDGE('',*,*,#13593,.T.);
#18075=ORIENTED_EDGE('',*,*,#13594,.T.);
#18076=ORIENTED_EDGE('',*,*,#13595,.T.);
#18077=ORIENTED_EDGE('',*,*,#13596,.T.);
#18078=ORIENTED_EDGE('',*,*,#13597,.T.);
#18079=ORIENTED_EDGE('',*,*,#13598,.T.);
#18080=ORIENTED_EDGE('',*,*,#13585,.F.);
#18081=ORIENTED_EDGE('',*,*,#13592,.T.);
#18082=ORIENTED_EDGE('',*,*,#13570,.F.);
#18083=ORIENTED_EDGE('',*,*,#13599,.T.);
#18084=ORIENTED_EDGE('',*,*,#13600,.T.);
#18085=ORIENTED_EDGE('',*,*,#13584,.F.);
#18086=ORIENTED_EDGE('',*,*,#13601,.F.);
#18087=ORIENTED_EDGE('',*,*,#13602,.T.);
#18088=ORIENTED_EDGE('',*,*,#13596,.F.);
#18089=ORIENTED_EDGE('',*,*,#13603,.T.);
#18090=ORIENTED_EDGE('',*,*,#13604,.F.);
#18091=ORIENTED_EDGE('',*,*,#13588,.F.);
#18092=ORIENTED_EDGE('',*,*,#13595,.F.);
#18093=ORIENTED_EDGE('',*,*,#13605,.F.);
#18094=ORIENTED_EDGE('',*,*,#13590,.F.);
#18095=ORIENTED_EDGE('',*,*,#13600,.F.);
#18096=ORIENTED_EDGE('',*,*,#13606,.F.);
#18097=ORIENTED_EDGE('',*,*,#13607,.F.);
#18098=ORIENTED_EDGE('',*,*,#13608,.F.);
#18099=ORIENTED_EDGE('',*,*,#13609,.F.);
#18100=ORIENTED_EDGE('',*,*,#13597,.F.);
#18101=ORIENTED_EDGE('',*,*,#13602,.F.);
#18102=ORIENTED_EDGE('',*,*,#13610,.F.);
#18103=ORIENTED_EDGE('',*,*,#13603,.F.);
#18104=ORIENTED_EDGE('',*,*,#13594,.F.);
#18105=ORIENTED_EDGE('',*,*,#13611,.F.);
#18106=ORIENTED_EDGE('',*,*,#13612,.T.);
#18107=ORIENTED_EDGE('',*,*,#13613,.T.);
#18108=ORIENTED_EDGE('',*,*,#13614,.T.);
#18109=ORIENTED_EDGE('',*,*,#13615,.T.);
#18110=ORIENTED_EDGE('',*,*,#13569,.F.);
#18111=ORIENTED_EDGE('',*,*,#13616,.F.);
#18112=ORIENTED_EDGE('',*,*,#13606,.T.);
#18113=ORIENTED_EDGE('',*,*,#13599,.F.);
#18114=ORIENTED_EDGE('',*,*,#13609,.T.);
#18115=ORIENTED_EDGE('',*,*,#13617,.F.);
#18116=ORIENTED_EDGE('',*,*,#13582,.F.);
#18117=ORIENTED_EDGE('',*,*,#13598,.F.);
#18118=ORIENTED_EDGE('',*,*,#13586,.F.);
#18119=ORIENTED_EDGE('',*,*,#13618,.F.);
#18120=ORIENTED_EDGE('',*,*,#13611,.T.);
#18121=ORIENTED_EDGE('',*,*,#13593,.F.);
#18122=ORIENTED_EDGE('',*,*,#13615,.F.);
#18123=ORIENTED_EDGE('',*,*,#13619,.F.);
#18124=ORIENTED_EDGE('',*,*,#13573,.F.);
#18125=ORIENTED_EDGE('',*,*,#13620,.F.);
#18126=ORIENTED_EDGE('',*,*,#13613,.F.);
#18127=ORIENTED_EDGE('',*,*,#13621,.F.);
#18128=ORIENTED_EDGE('',*,*,#13575,.F.);
#18129=ORIENTED_EDGE('',*,*,#13622,.F.);
#18130=ORIENTED_EDGE('',*,*,#13623,.F.);
#18131=ORIENTED_EDGE('',*,*,#13620,.T.);
#18132=ORIENTED_EDGE('',*,*,#13572,.F.);
#18133=ORIENTED_EDGE('',*,*,#13621,.T.);
#18134=ORIENTED_EDGE('',*,*,#13612,.F.);
#18135=ORIENTED_EDGE('',*,*,#13619,.T.);
#18136=ORIENTED_EDGE('',*,*,#13614,.F.);
#18137=ORIENTED_EDGE('',*,*,#13622,.T.);
#18138=ORIENTED_EDGE('',*,*,#13574,.F.);
#18139=ORIENTED_EDGE('',*,*,#13623,.T.);
#18140=ORIENTED_EDGE('',*,*,#13624,.T.);
#18141=ORIENTED_EDGE('',*,*,#13625,.F.);
#18142=ORIENTED_EDGE('',*,*,#13626,.F.);
#18143=ORIENTED_EDGE('',*,*,#13627,.F.);
#18144=ORIENTED_EDGE('',*,*,#13624,.F.);
#18145=ORIENTED_EDGE('',*,*,#13576,.F.);
#18146=ORIENTED_EDGE('',*,*,#13628,.T.);
#18147=ORIENTED_EDGE('',*,*,#13627,.T.);
#18148=ORIENTED_EDGE('',*,*,#13626,.T.);
#18149=ORIENTED_EDGE('',*,*,#13629,.T.);
#18150=ORIENTED_EDGE('',*,*,#13607,.T.);
#18151=ORIENTED_EDGE('',*,*,#13616,.T.);
#18152=ORIENTED_EDGE('',*,*,#13568,.T.);
#18153=ORIENTED_EDGE('',*,*,#13591,.T.);
#18154=ORIENTED_EDGE('',*,*,#13605,.T.);
#18155=ORIENTED_EDGE('',*,*,#13618,.T.);
#18156=ORIENTED_EDGE('',*,*,#13589,.T.);
#18157=ORIENTED_EDGE('',*,*,#13604,.T.);
#18158=ORIENTED_EDGE('',*,*,#13610,.T.);
#18159=ORIENTED_EDGE('',*,*,#13601,.T.);
#18160=ORIENTED_EDGE('',*,*,#13583,.T.);
#18161=ORIENTED_EDGE('',*,*,#13617,.T.);
#18162=ORIENTED_EDGE('',*,*,#13608,.T.);
#18163=ORIENTED_EDGE('',*,*,#13629,.F.);
#18164=ORIENTED_EDGE('',*,*,#13625,.T.);
#18165=ORIENTED_EDGE('',*,*,#13628,.F.);
#18166=ORIENTED_EDGE('',*,*,#13630,.T.);
#18167=ORIENTED_EDGE('',*,*,#13631,.T.);
#18168=ORIENTED_EDGE('',*,*,#13632,.T.);
#18169=ORIENTED_EDGE('',*,*,#13633,.T.);
#18170=ORIENTED_EDGE('',*,*,#13634,.T.);
#18171=ORIENTED_EDGE('',*,*,#13635,.T.);
#18172=ORIENTED_EDGE('',*,*,#13636,.T.);
#18173=ORIENTED_EDGE('',*,*,#13637,.T.);
#18174=ORIENTED_EDGE('',*,*,#13638,.T.);
#18175=ORIENTED_EDGE('',*,*,#13639,.T.);
#18176=ORIENTED_EDGE('',*,*,#13640,.T.);
#18177=ORIENTED_EDGE('',*,*,#13641,.T.);
#18178=ORIENTED_EDGE('',*,*,#13642,.T.);
#18179=ORIENTED_EDGE('',*,*,#13643,.T.);
#18180=ORIENTED_EDGE('',*,*,#13644,.T.);
#18181=ORIENTED_EDGE('',*,*,#13645,.T.);
#18182=ORIENTED_EDGE('',*,*,#13646,.T.);
#18183=ORIENTED_EDGE('',*,*,#13647,.T.);
#18184=ORIENTED_EDGE('',*,*,#13648,.T.);
#18185=ORIENTED_EDGE('',*,*,#13649,.T.);
#18186=ORIENTED_EDGE('',*,*,#13650,.T.);
#18187=ORIENTED_EDGE('',*,*,#13651,.T.);
#18188=ORIENTED_EDGE('',*,*,#13652,.T.);
#18189=ORIENTED_EDGE('',*,*,#13653,.T.);
#18190=ORIENTED_EDGE('',*,*,#13654,.T.);
#18191=ORIENTED_EDGE('',*,*,#13655,.T.);
#18192=ORIENTED_EDGE('',*,*,#13656,.T.);
#18193=ORIENTED_EDGE('',*,*,#13657,.T.);
#18194=ORIENTED_EDGE('',*,*,#13658,.T.);
#18195=ORIENTED_EDGE('',*,*,#13659,.T.);
#18196=ORIENTED_EDGE('',*,*,#13660,.T.);
#18197=ORIENTED_EDGE('',*,*,#13661,.T.);
#18198=ORIENTED_EDGE('',*,*,#13662,.T.);
#18199=ORIENTED_EDGE('',*,*,#13663,.T.);
#18200=ORIENTED_EDGE('',*,*,#13664,.T.);
#18201=ORIENTED_EDGE('',*,*,#13665,.T.);
#18202=ORIENTED_EDGE('',*,*,#13666,.T.);
#18203=ORIENTED_EDGE('',*,*,#13667,.T.);
#18204=ORIENTED_EDGE('',*,*,#13668,.T.);
#18205=ORIENTED_EDGE('',*,*,#13669,.T.);
#18206=ORIENTED_EDGE('',*,*,#13670,.T.);
#18207=ORIENTED_EDGE('',*,*,#13671,.T.);
#18208=ORIENTED_EDGE('',*,*,#13672,.T.);
#18209=ORIENTED_EDGE('',*,*,#13673,.T.);
#18210=ORIENTED_EDGE('',*,*,#13674,.T.);
#18211=ORIENTED_EDGE('',*,*,#13675,.T.);
#18212=ORIENTED_EDGE('',*,*,#13676,.T.);
#18213=ORIENTED_EDGE('',*,*,#13677,.T.);
#18214=ORIENTED_EDGE('',*,*,#13641,.F.);
#18215=ORIENTED_EDGE('',*,*,#13678,.F.);
#18216=ORIENTED_EDGE('',*,*,#13676,.F.);
#18217=ORIENTED_EDGE('',*,*,#13679,.T.);
#18218=ORIENTED_EDGE('',*,*,#13640,.F.);
#18219=ORIENTED_EDGE('',*,*,#13680,.F.);
#18220=ORIENTED_EDGE('',*,*,#13677,.F.);
#18221=ORIENTED_EDGE('',*,*,#13678,.T.);
#18222=ORIENTED_EDGE('',*,*,#13642,.F.);
#18223=ORIENTED_EDGE('',*,*,#13679,.F.);
#18224=ORIENTED_EDGE('',*,*,#13675,.F.);
#18225=ORIENTED_EDGE('',*,*,#13681,.T.);
#18226=ORIENTED_EDGE('',*,*,#13643,.F.);
#18227=ORIENTED_EDGE('',*,*,#13681,.F.);
#18228=ORIENTED_EDGE('',*,*,#13674,.F.);
#18229=ORIENTED_EDGE('',*,*,#13682,.T.);
#18230=ORIENTED_EDGE('',*,*,#13644,.F.);
#18231=ORIENTED_EDGE('',*,*,#13682,.F.);
#18232=ORIENTED_EDGE('',*,*,#13673,.F.);
#18233=ORIENTED_EDGE('',*,*,#13683,.T.);
#18234=ORIENTED_EDGE('',*,*,#13645,.F.);
#18235=ORIENTED_EDGE('',*,*,#13683,.F.);
#18236=ORIENTED_EDGE('',*,*,#13672,.F.);
#18237=ORIENTED_EDGE('',*,*,#13684,.T.);
#18238=ORIENTED_EDGE('',*,*,#13646,.F.);
#18239=ORIENTED_EDGE('',*,*,#13684,.F.);
#18240=ORIENTED_EDGE('',*,*,#13671,.F.);
#18241=ORIENTED_EDGE('',*,*,#13685,.T.);
#18242=ORIENTED_EDGE('',*,*,#13639,.F.);
#18243=ORIENTED_EDGE('',*,*,#13685,.F.);
#18244=ORIENTED_EDGE('',*,*,#13670,.F.);
#18245=ORIENTED_EDGE('',*,*,#13680,.T.);
#18246=ORIENTED_EDGE('',*,*,#13655,.F.);
#18247=ORIENTED_EDGE('',*,*,#13686,.F.);
#18248=ORIENTED_EDGE('',*,*,#13687,.F.);
#18249=ORIENTED_EDGE('',*,*,#13688,.T.);
#18250=ORIENTED_EDGE('',*,*,#13654,.F.);
#18251=ORIENTED_EDGE('',*,*,#13689,.F.);
#18252=ORIENTED_EDGE('',*,*,#13690,.F.);
#18253=ORIENTED_EDGE('',*,*,#13686,.T.);
#18254=ORIENTED_EDGE('',*,*,#13653,.F.);
#18255=ORIENTED_EDGE('',*,*,#13691,.F.);
#18256=ORIENTED_EDGE('',*,*,#13692,.F.);
#18257=ORIENTED_EDGE('',*,*,#13689,.T.);
#18258=ORIENTED_EDGE('',*,*,#13662,.F.);
#18259=ORIENTED_EDGE('',*,*,#13693,.F.);
#18260=ORIENTED_EDGE('',*,*,#13694,.F.);
#18261=ORIENTED_EDGE('',*,*,#13695,.T.);
#18262=ORIENTED_EDGE('',*,*,#13661,.F.);
#18263=ORIENTED_EDGE('',*,*,#13696,.F.);
#18264=ORIENTED_EDGE('',*,*,#13697,.F.);
#18265=ORIENTED_EDGE('',*,*,#13693,.T.);
#18266=ORIENTED_EDGE('',*,*,#13660,.F.);
#18267=ORIENTED_EDGE('',*,*,#13698,.F.);
#18268=ORIENTED_EDGE('',*,*,#13699,.F.);
#18269=ORIENTED_EDGE('',*,*,#13696,.T.);
#18270=ORIENTED_EDGE('',*,*,#13659,.F.);
#18271=ORIENTED_EDGE('',*,*,#13700,.F.);
#18272=ORIENTED_EDGE('',*,*,#13701,.F.);
#18273=ORIENTED_EDGE('',*,*,#13698,.T.);
#18274=ORIENTED_EDGE('',*,*,#13658,.F.);
#18275=ORIENTED_EDGE('',*,*,#13702,.F.);
#18276=ORIENTED_EDGE('',*,*,#13703,.F.);
#18277=ORIENTED_EDGE('',*,*,#13700,.T.);
#18278=ORIENTED_EDGE('',*,*,#13657,.F.);
#18279=ORIENTED_EDGE('',*,*,#13704,.F.);
#18280=ORIENTED_EDGE('',*,*,#13705,.F.);
#18281=ORIENTED_EDGE('',*,*,#13702,.T.);
#18282=ORIENTED_EDGE('',*,*,#13656,.F.);
#18283=ORIENTED_EDGE('',*,*,#13688,.F.);
#18284=ORIENTED_EDGE('',*,*,#13706,.F.);
#18285=ORIENTED_EDGE('',*,*,#13704,.T.);
#18286=ORIENTED_EDGE('',*,*,#13663,.F.);
#18287=ORIENTED_EDGE('',*,*,#13695,.F.);
#18288=ORIENTED_EDGE('',*,*,#13707,.F.);
#18289=ORIENTED_EDGE('',*,*,#13691,.T.);
#18290=ORIENTED_EDGE('',*,*,#13692,.T.);
#18291=ORIENTED_EDGE('',*,*,#13707,.T.);
#18292=ORIENTED_EDGE('',*,*,#13694,.T.);
#18293=ORIENTED_EDGE('',*,*,#13697,.T.);
#18294=ORIENTED_EDGE('',*,*,#13699,.T.);
#18295=ORIENTED_EDGE('',*,*,#13701,.T.);
#18296=ORIENTED_EDGE('',*,*,#13703,.T.);
#18297=ORIENTED_EDGE('',*,*,#13705,.T.);
#18298=ORIENTED_EDGE('',*,*,#13706,.T.);
#18299=ORIENTED_EDGE('',*,*,#13687,.T.);
#18300=ORIENTED_EDGE('',*,*,#13690,.T.);
#18301=ORIENTED_EDGE('',*,*,#13708,.T.);
#18302=ORIENTED_EDGE('',*,*,#13709,.T.);
#18303=ORIENTED_EDGE('',*,*,#13710,.T.);
#18304=ORIENTED_EDGE('',*,*,#13711,.T.);
#18305=ORIENTED_EDGE('',*,*,#13712,.T.);
#18306=ORIENTED_EDGE('',*,*,#13713,.T.);
#18307=ORIENTED_EDGE('',*,*,#13649,.F.);
#18308=ORIENTED_EDGE('',*,*,#13714,.F.);
#18309=ORIENTED_EDGE('',*,*,#13710,.F.);
#18310=ORIENTED_EDGE('',*,*,#13715,.T.);
#18311=ORIENTED_EDGE('',*,*,#13648,.F.);
#18312=ORIENTED_EDGE('',*,*,#13716,.F.);
#18313=ORIENTED_EDGE('',*,*,#13711,.F.);
#18314=ORIENTED_EDGE('',*,*,#13714,.T.);
#18315=ORIENTED_EDGE('',*,*,#13650,.F.);
#18316=ORIENTED_EDGE('',*,*,#13715,.F.);
#18317=ORIENTED_EDGE('',*,*,#13709,.F.);
#18318=ORIENTED_EDGE('',*,*,#13717,.T.);
#18319=ORIENTED_EDGE('',*,*,#13651,.F.);
#18320=ORIENTED_EDGE('',*,*,#13717,.F.);
#18321=ORIENTED_EDGE('',*,*,#13708,.F.);
#18322=ORIENTED_EDGE('',*,*,#13718,.T.);
#18323=ORIENTED_EDGE('',*,*,#13652,.F.);
#18324=ORIENTED_EDGE('',*,*,#13718,.F.);
#18325=ORIENTED_EDGE('',*,*,#13713,.F.);
#18326=ORIENTED_EDGE('',*,*,#13719,.T.);
#18327=ORIENTED_EDGE('',*,*,#13647,.F.);
#18328=ORIENTED_EDGE('',*,*,#13719,.F.);
#18329=ORIENTED_EDGE('',*,*,#13712,.F.);
#18330=ORIENTED_EDGE('',*,*,#13716,.T.);
#18331=ORIENTED_EDGE('',*,*,#13668,.F.);
#18332=ORIENTED_EDGE('',*,*,#13720,.F.);
#18333=ORIENTED_EDGE('',*,*,#13721,.F.);
#18334=ORIENTED_EDGE('',*,*,#13722,.T.);
#18335=ORIENTED_EDGE('',*,*,#13667,.F.);
#18336=ORIENTED_EDGE('',*,*,#13723,.F.);
#18337=ORIENTED_EDGE('',*,*,#13724,.F.);
#18338=ORIENTED_EDGE('',*,*,#13720,.T.);
#18339=ORIENTED_EDGE('',*,*,#13666,.F.);
#18340=ORIENTED_EDGE('',*,*,#13725,.F.);
#18341=ORIENTED_EDGE('',*,*,#13726,.F.);
#18342=ORIENTED_EDGE('',*,*,#13723,.T.);
#18343=ORIENTED_EDGE('',*,*,#13665,.F.);
#18344=ORIENTED_EDGE('',*,*,#13727,.F.);
#18345=ORIENTED_EDGE('',*,*,#13728,.F.);
#18346=ORIENTED_EDGE('',*,*,#13725,.T.);
#18347=ORIENTED_EDGE('',*,*,#13669,.F.);
#18348=ORIENTED_EDGE('',*,*,#13722,.F.);
#18349=ORIENTED_EDGE('',*,*,#13729,.F.);
#18350=ORIENTED_EDGE('',*,*,#13730,.T.);
#18351=ORIENTED_EDGE('',*,*,#13664,.F.);
#18352=ORIENTED_EDGE('',*,*,#13730,.F.);
#18353=ORIENTED_EDGE('',*,*,#13731,.F.);
#18354=ORIENTED_EDGE('',*,*,#13727,.T.);
#18355=ORIENTED_EDGE('',*,*,#13726,.T.);
#18356=ORIENTED_EDGE('',*,*,#13728,.T.);
#18357=ORIENTED_EDGE('',*,*,#13731,.T.);
#18358=ORIENTED_EDGE('',*,*,#13729,.T.);
#18359=ORIENTED_EDGE('',*,*,#13721,.T.);
#18360=ORIENTED_EDGE('',*,*,#13724,.T.);
#18361=ORIENTED_EDGE('',*,*,#13633,.F.);
#18362=ORIENTED_EDGE('',*,*,#13732,.F.);
#18363=ORIENTED_EDGE('',*,*,#13733,.F.);
#18364=ORIENTED_EDGE('',*,*,#13734,.T.);
#18365=ORIENTED_EDGE('',*,*,#13632,.F.);
#18366=ORIENTED_EDGE('',*,*,#13735,.F.);
#18367=ORIENTED_EDGE('',*,*,#13736,.F.);
#18368=ORIENTED_EDGE('',*,*,#13732,.T.);
#18369=ORIENTED_EDGE('',*,*,#13631,.F.);
#18370=ORIENTED_EDGE('',*,*,#13737,.F.);
#18371=ORIENTED_EDGE('',*,*,#13738,.F.);
#18372=ORIENTED_EDGE('',*,*,#13735,.T.);
#18373=ORIENTED_EDGE('',*,*,#13630,.F.);
#18374=ORIENTED_EDGE('',*,*,#13739,.F.);
#18375=ORIENTED_EDGE('',*,*,#13740,.F.);
#18376=ORIENTED_EDGE('',*,*,#13737,.T.);
#18377=ORIENTED_EDGE('',*,*,#13638,.F.);
#18378=ORIENTED_EDGE('',*,*,#13741,.F.);
#18379=ORIENTED_EDGE('',*,*,#13742,.F.);
#18380=ORIENTED_EDGE('',*,*,#13739,.T.);
#18381=ORIENTED_EDGE('',*,*,#13581,.F.);
#18382=ORIENTED_EDGE('',*,*,#13743,.F.);
#18383=ORIENTED_EDGE('',*,*,#13744,.F.);
#18384=ORIENTED_EDGE('',*,*,#13745,.T.);
#18385=ORIENTED_EDGE('',*,*,#13580,.F.);
#18386=ORIENTED_EDGE('',*,*,#13746,.F.);
#18387=ORIENTED_EDGE('',*,*,#13747,.F.);
#18388=ORIENTED_EDGE('',*,*,#13743,.T.);
#18389=ORIENTED_EDGE('',*,*,#13637,.F.);
#18390=ORIENTED_EDGE('',*,*,#13748,.F.);
#18391=ORIENTED_EDGE('',*,*,#13749,.F.);
#18392=ORIENTED_EDGE('',*,*,#13741,.T.);
#18393=ORIENTED_EDGE('',*,*,#13636,.F.);
#18394=ORIENTED_EDGE('',*,*,#13750,.F.);
#18395=ORIENTED_EDGE('',*,*,#13751,.F.);
#18396=ORIENTED_EDGE('',*,*,#13748,.T.);
#18397=ORIENTED_EDGE('',*,*,#13635,.F.);
#18398=ORIENTED_EDGE('',*,*,#13752,.F.);
#18399=ORIENTED_EDGE('',*,*,#13753,.F.);
#18400=ORIENTED_EDGE('',*,*,#13750,.T.);
#18401=ORIENTED_EDGE('',*,*,#13634,.F.);
#18402=ORIENTED_EDGE('',*,*,#13734,.F.);
#18403=ORIENTED_EDGE('',*,*,#13754,.F.);
#18404=ORIENTED_EDGE('',*,*,#13752,.T.);
#18405=ORIENTED_EDGE('',*,*,#13579,.F.);
#18406=ORIENTED_EDGE('',*,*,#13755,.F.);
#18407=ORIENTED_EDGE('',*,*,#13756,.F.);
#18408=ORIENTED_EDGE('',*,*,#13746,.T.);
#18409=ORIENTED_EDGE('',*,*,#13578,.F.);
#18410=ORIENTED_EDGE('',*,*,#13745,.F.);
#18411=ORIENTED_EDGE('',*,*,#13757,.F.);
#18412=ORIENTED_EDGE('',*,*,#13755,.T.);
#18413=ORIENTED_EDGE('',*,*,#13740,.T.);
#18414=ORIENTED_EDGE('',*,*,#13742,.T.);
#18415=ORIENTED_EDGE('',*,*,#13749,.T.);
#18416=ORIENTED_EDGE('',*,*,#13751,.T.);
#18417=ORIENTED_EDGE('',*,*,#13753,.T.);
#18418=ORIENTED_EDGE('',*,*,#13754,.T.);
#18419=ORIENTED_EDGE('',*,*,#13733,.T.);
#18420=ORIENTED_EDGE('',*,*,#13736,.T.);
#18421=ORIENTED_EDGE('',*,*,#13738,.T.);
#18422=ORIENTED_EDGE('',*,*,#13747,.T.);
#18423=ORIENTED_EDGE('',*,*,#13756,.T.);
#18424=ORIENTED_EDGE('',*,*,#13757,.T.);
#18425=ORIENTED_EDGE('',*,*,#13744,.T.);
#22846=CYLINDRICAL_SURFACE('',#25668,20.);
#22847=CYLINDRICAL_SURFACE('',#25680,11.5);
#22848=CYLINDRICAL_SURFACE('',#25682,12.);
#22849=CYLINDRICAL_SURFACE('',#25684,12.);
#22850=CYLINDRICAL_SURFACE('',#25686,12.);
#22851=CYLINDRICAL_SURFACE('',#25688,11.5);
#22852=CYLINDRICAL_SURFACE('',#25690,11.5);
#22853=CYLINDRICAL_SURFACE('',#25701,11.5);
#22854=CYLINDRICAL_SURFACE('',#25702,11.5);
#22855=CYLINDRICAL_SURFACE('',#25703,11.5);
#22856=CYLINDRICAL_SURFACE('',#25704,7.);
#22857=CYLINDRICAL_SURFACE('',#25709,2.1);
#22858=CYLINDRICAL_SURFACE('',#25710,20.);
#22859=CYLINDRICAL_SURFACE('',#25734,19.5);
#22860=CYLINDRICAL_SURFACE('',#25765,19.5);
#22861=CYLINDRICAL_SURFACE('',#25766,19.5);
#22862=CYLINDRICAL_SURFACE('',#25787,19.5);
#22863=CYLINDRICAL_SURFACE('',#25793,1.4361111111);
#22864=CYLINDRICAL_SURFACE('',#25804,0.4033333333);
#22865=CYLINDRICAL_SURFACE('',#25806,19.5);
#23624=ADVANCED_FACE('',(#2632),#1550,.T.);
#23625=ADVANCED_FACE('',(#2633,#1139),#1551,.T.);
#23626=ADVANCED_FACE('',(#2634),#2122,.T.);
#23627=ADVANCED_FACE('',(#2635),#22846,.T.);
#23628=ADVANCED_FACE('',(#2636),#1552,.T.);
#23629=ADVANCED_FACE('',(#2637),#1553,.T.);
#23630=ADVANCED_FACE('',(#2638),#22847,.F.);
#23631=ADVANCED_FACE('',(#2639),#22848,.F.);
#23632=ADVANCED_FACE('',(#2640),#22849,.F.);
#23633=ADVANCED_FACE('',(#2641),#22850,.F.);
#23634=ADVANCED_FACE('',(#2642),#22851,.F.);
#23635=ADVANCED_FACE('',(#2643),#22852,.F.);
#23636=ADVANCED_FACE('',(#2644,#1140),#1554,.F.);
#23637=ADVANCED_FACE('',(#2645),#22853,.F.);
#23638=ADVANCED_FACE('',(#2646),#22854,.F.);
#23639=ADVANCED_FACE('',(#2647),#22855,.F.);
#23640=ADVANCED_FACE('',(#2648),#22856,.F.);
#23641=ADVANCED_FACE('',(#2649,#1141),#1555,.F.);
#23642=ADVANCED_FACE('',(#2650),#1556,.T.);
#23643=ADVANCED_FACE('',(#2651),#1557,.T.);
#23644=ADVANCED_FACE('',(#2652),#22857,.F.);
#23645=ADVANCED_FACE('',(#2653,#1142,#1143,#1144,#1145,#1146),#22858,.T.);
#23646=ADVANCED_FACE('',(#2654),#22859,.T.);
#23647=ADVANCED_FACE('',(#2655),#1558,.F.);
#23648=ADVANCED_FACE('',(#2656),#1559,.F.);
#23649=ADVANCED_FACE('',(#2657),#1560,.F.);
#23650=ADVANCED_FACE('',(#2658),#1561,.F.);
#23651=ADVANCED_FACE('',(#2659),#1562,.F.);
#23652=ADVANCED_FACE('',(#2660),#1563,.F.);
#23653=ADVANCED_FACE('',(#2661),#1564,.F.);
#23654=ADVANCED_FACE('',(#2662),#1565,.F.);
#23655=ADVANCED_FACE('',(#2663),#1566,.F.);
#23656=ADVANCED_FACE('',(#2664),#1567,.F.);
#23657=ADVANCED_FACE('',(#2665),#1568,.F.);
#23658=ADVANCED_FACE('',(#2666),#1569,.F.);
#23659=ADVANCED_FACE('',(#2667),#1570,.F.);
#23660=ADVANCED_FACE('',(#2668),#1571,.F.);
#23661=ADVANCED_FACE('',(#2669),#1572,.F.);
#23662=ADVANCED_FACE('',(#2670),#1573,.F.);
#23663=ADVANCED_FACE('',(#2671),#1574,.F.);
#23664=ADVANCED_FACE('',(#2672),#1575,.F.);
#23665=ADVANCED_FACE('',(#2673),#1576,.F.);
#23666=ADVANCED_FACE('',(#2674),#22860,.T.);
#23667=ADVANCED_FACE('',(#2675),#22861,.T.);
#23668=ADVANCED_FACE('',(#2676),#1577,.F.);
#23669=ADVANCED_FACE('',(#2677),#1578,.F.);
#23670=ADVANCED_FACE('',(#2678),#1579,.F.);
#23671=ADVANCED_FACE('',(#2679),#1580,.F.);
#23672=ADVANCED_FACE('',(#2680),#1581,.F.);
#23673=ADVANCED_FACE('',(#2681),#1582,.F.);
#23674=ADVANCED_FACE('',(#2682),#1583,.F.);
#23675=ADVANCED_FACE('',(#2683),#1584,.F.);
#23676=ADVANCED_FACE('',(#2684),#1585,.F.);
#23677=ADVANCED_FACE('',(#2685),#1586,.F.);
#23678=ADVANCED_FACE('',(#2686),#1587,.F.);
#23679=ADVANCED_FACE('',(#2687),#1588,.F.);
#23680=ADVANCED_FACE('',(#2688),#22862,.T.);
#23681=ADVANCED_FACE('',(#2689),#1589,.F.);
#23682=ADVANCED_FACE('',(#2690),#1590,.F.);
#23683=ADVANCED_FACE('',(#2691),#1591,.F.);
#23684=ADVANCED_FACE('',(#2692),#22863,.F.);
#23685=ADVANCED_FACE('',(#2693),#1592,.F.);
#23686=ADVANCED_FACE('',(#2694),#1593,.T.);
#23687=ADVANCED_FACE('',(#2695),#1594,.T.);
#23688=ADVANCED_FACE('',(#2696),#1595,.F.);
#23689=ADVANCED_FACE('',(#2697),#1596,.F.);
#23690=ADVANCED_FACE('',(#2698),#1597,.F.);
#23691=ADVANCED_FACE('',(#2699),#1598,.F.);
#23692=ADVANCED_FACE('',(#2700),#22864,.T.);
#23693=ADVANCED_FACE('',(#2701),#1599,.T.);
#23694=ADVANCED_FACE('',(#2702,#1147),#22865,.T.);
#24541=CLOSED_SHELL('',(#23624,#23625,#23626,#23627,#23628,#23629,#23630,
#23631,#23632,#23633,#23634,#23635,#23636,#23637,#23638,#23639,#23640,#23641,
#23642,#23643,#23644,#23645,#23646,#23647,#23648,#23649,#23650,#23651,#23652,
#23653,#23654,#23655,#23656,#23657,#23658,#23659,#23660,#23661,#23662,#23663,
#23664,#23665,#23666,#23667,#23668,#23669,#23670,#23671,#23672,#23673,#23674,
#23675,#23676,#23677,#23678,#23679,#23680,#23681,#23682,#23683,#23684,#23685,
#23686,#23687,#23688,#23689,#23690,#23691,#23692,#23693,#23694));
#25657=AXIS2_PLACEMENT_3D('',#51705,#29513,#29514);
#25658=AXIS2_PLACEMENT_3D('',#51706,#29515,#29516);
#25659=AXIS2_PLACEMENT_3D('',#51709,#29517,#29518);
#25660=AXIS2_PLACEMENT_3D('',#51711,#29519,#29520);
#25661=AXIS2_PLACEMENT_3D('',#51713,#29521,#29522);
#25662=AXIS2_PLACEMENT_3D('',#51714,#29523,#29524);
#25663=AXIS2_PLACEMENT_3D('',#51715,#29525,#29526);
#25664=AXIS2_PLACEMENT_3D('',#51717,#29527,#29528);
#25665=AXIS2_PLACEMENT_3D('',#51722,#29530,#29531);
#25666=AXIS2_PLACEMENT_3D('',#51726,#29534,#29535);
#25667=AXIS2_PLACEMENT_3D('',#51728,#29536,#29537);
#25668=AXIS2_PLACEMENT_3D('',#51730,#29539,#29540);
#25669=AXIS2_PLACEMENT_3D('',#51755,#29543,#29544);
#25670=AXIS2_PLACEMENT_3D('',#51756,#29545,#29546);
#25671=AXIS2_PLACEMENT_3D('',#51759,#29547,#29548);
#25672=AXIS2_PLACEMENT_3D('',#51761,#29549,#29550);
#25673=AXIS2_PLACEMENT_3D('',#51763,#29551,#29552);
#25674=AXIS2_PLACEMENT_3D('',#51764,#29553,#29554);
#25675=AXIS2_PLACEMENT_3D('',#51765,#29555,#29556);
#25676=AXIS2_PLACEMENT_3D('',#51768,#29557,#29558);
#25677=AXIS2_PLACEMENT_3D('',#51770,#29559,#29560);
#25678=AXIS2_PLACEMENT_3D('',#51772,#29561,#29562);
#25679=AXIS2_PLACEMENT_3D('',#51773,#29563,#29564);
#25680=AXIS2_PLACEMENT_3D('',#51774,#29565,#29566);
#25681=AXIS2_PLACEMENT_3D('',#51777,#29567,#29568);
#25682=AXIS2_PLACEMENT_3D('',#51780,#29571,#29572);
#25683=AXIS2_PLACEMENT_3D('',#51784,#29574,#29575);
#25684=AXIS2_PLACEMENT_3D('',#51786,#29577,#29578);
#25685=AXIS2_PLACEMENT_3D('',#51790,#29580,#29581);
#25686=AXIS2_PLACEMENT_3D('',#51792,#29583,#29584);
#25687=AXIS2_PLACEMENT_3D('',#51795,#29586,#29587);
#25688=AXIS2_PLACEMENT_3D('',#51796,#29588,#29589);
#25689=AXIS2_PLACEMENT_3D('',#51799,#29591,#29592);
#25690=AXIS2_PLACEMENT_3D('',#51800,#29593,#29594);
#25691=AXIS2_PLACEMENT_3D('',#51802,#29595,#29596);
#25692=AXIS2_PLACEMENT_3D('',#51804,#29598,#29599);
#25693=AXIS2_PLACEMENT_3D('',#51806,#29600,#29601);
#25694=AXIS2_PLACEMENT_3D('',#51808,#29602,#29603);
#25695=AXIS2_PLACEMENT_3D('',#51810,#29604,#29605);
#25696=AXIS2_PLACEMENT_3D('',#51812,#29606,#29607);
#25697=AXIS2_PLACEMENT_3D('',#51813,#29608,#29609);
#25698=AXIS2_PLACEMENT_3D('',#51814,#29610,#29611);
#25699=AXIS2_PLACEMENT_3D('',#51815,#29612,#29613);
#25700=AXIS2_PLACEMENT_3D('',#51823,#29617,#29618);
#25701=AXIS2_PLACEMENT_3D('',#51824,#29619,#29620);
#25702=AXIS2_PLACEMENT_3D('',#51826,#29622,#29623);
#25703=AXIS2_PLACEMENT_3D('',#51828,#29625,#29626);
#25704=AXIS2_PLACEMENT_3D('',#51830,#29628,#29629);
#25705=AXIS2_PLACEMENT_3D('',#51833,#29632,#29633);
#25706=AXIS2_PLACEMENT_3D('',#51837,#29636,#29637);
#25707=AXIS2_PLACEMENT_3D('',#51838,#29638,#29639);
#25708=AXIS2_PLACEMENT_3D('',#51839,#29640,#29641);
#25709=AXIS2_PLACEMENT_3D('',#51840,#29642,#29643);
#25710=AXIS2_PLACEMENT_3D('',#51883,#29645,#29646);
#25711=AXIS2_PLACEMENT_3D('',#51905,#29649,#29650);
#25712=AXIS2_PLACEMENT_3D('',#51909,#29652,#29653);
#25713=AXIS2_PLACEMENT_3D('',#51913,#29655,#29656);
#25714=AXIS2_PLACEMENT_3D('',#51917,#29658,#29659);
#25715=AXIS2_PLACEMENT_3D('',#51921,#29661,#29662);
#25716=AXIS2_PLACEMENT_3D('',#51925,#29664,#29665);
#25717=AXIS2_PLACEMENT_3D('',#51929,#29667,#29668);
#25718=AXIS2_PLACEMENT_3D('',#51933,#29670,#29671);
#25719=AXIS2_PLACEMENT_3D('',#51939,#29674,#29675);
#25720=AXIS2_PLACEMENT_3D('',#51941,#29676,#29677);
#25721=AXIS2_PLACEMENT_3D('',#51945,#29679,#29680);
#25722=AXIS2_PLACEMENT_3D('',#51946,#29681,#29682);
#25723=AXIS2_PLACEMENT_3D('',#51949,#29683,#29684);
#25724=AXIS2_PLACEMENT_3D('',#51953,#29686,#29687);
#25725=AXIS2_PLACEMENT_3D('',#51955,#29688,#29689);
#25726=AXIS2_PLACEMENT_3D('',#51959,#29691,#29692);
#25727=AXIS2_PLACEMENT_3D('',#51963,#29694,#29695);
#25728=AXIS2_PLACEMENT_3D('',#51965,#29696,#29697);
#25729=AXIS2_PLACEMENT_3D('',#51968,#29699,#29700);
#25730=AXIS2_PLACEMENT_3D('',#51971,#29701,#29702);
#25731=AXIS2_PLACEMENT_3D('',#51975,#29704,#29705);
#25732=AXIS2_PLACEMENT_3D('',#51977,#29706,#29707);
#25733=AXIS2_PLACEMENT_3D('',#51980,#29709,#29710);
#25734=AXIS2_PLACEMENT_3D('',#51981,#29711,#29712);
#25735=AXIS2_PLACEMENT_3D('',#51984,#29713,#29714);
#25736=AXIS2_PLACEMENT_3D('',#51988,#29716,#29717);
#25737=AXIS2_PLACEMENT_3D('',#51992,#29719,#29720);
#25738=AXIS2_PLACEMENT_3D('',#51996,#29722,#29723);
#25739=AXIS2_PLACEMENT_3D('',#51998,#29725,#29726);
#25740=AXIS2_PLACEMENT_3D('',#52001,#29729,#29730);
#25741=AXIS2_PLACEMENT_3D('',#52003,#29732,#29733);
#25742=AXIS2_PLACEMENT_3D('',#52005,#29735,#29736);
#25743=AXIS2_PLACEMENT_3D('',#52007,#29738,#29739);
#25744=AXIS2_PLACEMENT_3D('',#52009,#29741,#29742);
#25745=AXIS2_PLACEMENT_3D('',#52011,#29744,#29745);
#25746=AXIS2_PLACEMENT_3D('',#52013,#29747,#29748);
#25747=AXIS2_PLACEMENT_3D('',#52014,#29749,#29750);
#25748=AXIS2_PLACEMENT_3D('',#52018,#29752,#29753);
#25749=AXIS2_PLACEMENT_3D('',#52020,#29755,#29756);
#25750=AXIS2_PLACEMENT_3D('',#52024,#29759,#29760);
#25751=AXIS2_PLACEMENT_3D('',#52027,#29762,#29763);
#25752=AXIS2_PLACEMENT_3D('',#52028,#29764,#29765);
#25753=AXIS2_PLACEMENT_3D('',#52034,#29769,#29770);
#25754=AXIS2_PLACEMENT_3D('',#52037,#29772,#29773);
#25755=AXIS2_PLACEMENT_3D('',#52038,#29774,#29775);
#25756=AXIS2_PLACEMENT_3D('',#52041,#29777,#29778);
#25757=AXIS2_PLACEMENT_3D('',#52042,#29779,#29780);
#25758=AXIS2_PLACEMENT_3D('',#52046,#29783,#29784);
#25759=AXIS2_PLACEMENT_3D('',#52049,#29786,#29787);
#25760=AXIS2_PLACEMENT_3D('',#52050,#29788,#29789);
#25761=AXIS2_PLACEMENT_3D('',#52054,#29792,#29793);
#25762=AXIS2_PLACEMENT_3D('',#52055,#29794,#29795);
#25763=AXIS2_PLACEMENT_3D('',#52056,#29796,#29797);
#25764=AXIS2_PLACEMENT_3D('',#52057,#29798,#29799);
#25765=AXIS2_PLACEMENT_3D('',#52058,#29800,#29801);
#25766=AXIS2_PLACEMENT_3D('',#52059,#29802,#29803);
#25767=AXIS2_PLACEMENT_3D('',#52062,#29804,#29805);
#25768=AXIS2_PLACEMENT_3D('',#52066,#29807,#29808);
#25769=AXIS2_PLACEMENT_3D('',#52068,#29809,#29810);
#25770=AXIS2_PLACEMENT_3D('',#52071,#29812,#29813);
#25771=AXIS2_PLACEMENT_3D('',#52072,#29814,#29815);
#25772=AXIS2_PLACEMENT_3D('',#52075,#29818,#29819);
#25773=AXIS2_PLACEMENT_3D('',#52077,#29821,#29822);
#25774=AXIS2_PLACEMENT_3D('',#52079,#29824,#29825);
#25775=AXIS2_PLACEMENT_3D('',#52081,#29827,#29828);
#25776=AXIS2_PLACEMENT_3D('',#52083,#29830,#29831);
#25777=AXIS2_PLACEMENT_3D('',#52084,#29832,#29833);
#25778=AXIS2_PLACEMENT_3D('',#52090,#29837,#29838);
#25779=AXIS2_PLACEMENT_3D('',#52093,#29840,#29841);
#25780=AXIS2_PLACEMENT_3D('',#52094,#29842,#29843);
#25781=AXIS2_PLACEMENT_3D('',#52097,#29845,#29846);
#25782=AXIS2_PLACEMENT_3D('',#52098,#29847,#29848);
#25783=AXIS2_PLACEMENT_3D('',#52102,#29851,#29852);
#25784=AXIS2_PLACEMENT_3D('',#52104,#29853,#29854);
#25785=AXIS2_PLACEMENT_3D('',#52106,#29856,#29857);
#25786=AXIS2_PLACEMENT_3D('',#52107,#29858,#29859);
#25787=AXIS2_PLACEMENT_3D('',#52108,#29860,#29861);
#25788=AXIS2_PLACEMENT_3D('',#52109,#29862,#29863);
#25789=AXIS2_PLACEMENT_3D('',#52113,#29865,#29866);
#25790=AXIS2_PLACEMENT_3D('',#52115,#29868,#29869);
#25791=AXIS2_PLACEMENT_3D('',#52119,#29872,#29873);
#25792=AXIS2_PLACEMENT_3D('',#52122,#29875,#29876);
#25793=AXIS2_PLACEMENT_3D('',#52123,#29877,#29878);
#25794=AXIS2_PLACEMENT_3D('',#52142,#29880,#29881);
#25795=AXIS2_PLACEMENT_3D('',#52146,#29884,#29885);
#25796=AXIS2_PLACEMENT_3D('',#52150,#29887,#29888);
#25797=AXIS2_PLACEMENT_3D('',#52152,#29890,#29891);
#25798=AXIS2_PLACEMENT_3D('',#52156,#29894,#29895);
#25799=AXIS2_PLACEMENT_3D('',#52159,#29897,#29898);
#25800=AXIS2_PLACEMENT_3D('',#52160,#29899,#29900);
#25801=AXIS2_PLACEMENT_3D('',#52164,#29903,#29904);
#25802=AXIS2_PLACEMENT_3D('',#52167,#29906,#29907);
#25803=AXIS2_PLACEMENT_3D('',#52168,#29908,#29909);
#25804=AXIS2_PLACEMENT_3D('',#52170,#29911,#29912);
#25805=AXIS2_PLACEMENT_3D('',#52191,#29914,#29915);
#25806=AXIS2_PLACEMENT_3D('',#52193,#29917,#29918);
#29513=DIRECTION('axis',(0.,0.,1.));
#29514=DIRECTION('refdir',(1.,0.,0.));
#29515=DIRECTION('center_axis',(-1.,0.,0.));
#29516=DIRECTION('ref_axis',(0.,0.,1.));
#29517=DIRECTION('center_axis',(1.,0.,0.));
#29518=DIRECTION('ref_axis',(0.,-0.499999999993262,0.866025403788329));
#29519=DIRECTION('center_axis',(1.,0.,0.));
#29520=DIRECTION('ref_axis',(0.,0.,-1.));
#29521=DIRECTION('center_axis',(1.,0.,0.));
#29522=DIRECTION('ref_axis',(0.,1.,0.));
#29523=DIRECTION('center_axis',(1.,0.,0.));
#29524=DIRECTION('ref_axis',(0.,0.,1.));
#29525=DIRECTION('center_axis',(1.,0.,0.));
#29526=DIRECTION('ref_axis',(0.,1.,0.));
#29527=DIRECTION('center_axis',(1.,0.,0.));
#29528=DIRECTION('ref_axis',(0.,0.,-1.));
#29529=DIRECTION('',(0.,0.,-1.));
#29530=DIRECTION('center_axis',(-1.,0.,0.));
#29531=DIRECTION('ref_axis',(0.,0.,-1.));
#29532=DIRECTION('',(0.,0.,1.));
#29533=DIRECTION('',(0.,1.,0.));
#29534=DIRECTION('center_axis',(-1.,0.,0.));
#29535=DIRECTION('ref_axis',(0.,0.,-1.));
#29536=DIRECTION('center_axis',(1.,0.,0.));
#29537=DIRECTION('ref_axis',(0.,0.,-1.));
#29538=DIRECTION('',(0.707106781186548,-8.65956056235493E-17,-0.707106781186547));
#29539=DIRECTION('center_axis',(1.,0.,0.));
#29540=DIRECTION('ref_axis',(0.,0.,-1.));
#29541=DIRECTION('',(1.,0.,0.));
#29542=DIRECTION('',(-1.,0.,0.));
#29543=DIRECTION('center_axis',(1.,0.,0.));
#29544=DIRECTION('ref_axis',(0.,0.,-1.));
#29545=DIRECTION('center_axis',(-1.,0.,0.));
#29546=DIRECTION('ref_axis',(0.,0.,1.));
#29547=DIRECTION('center_axis',(1.,0.,0.));
#29548=DIRECTION('ref_axis',(0.,1.,0.));
#29549=DIRECTION('center_axis',(1.,0.,0.));
#29550=DIRECTION('ref_axis',(0.,0.,-1.));
#29551=DIRECTION('center_axis',(1.,0.,0.));
#29552=DIRECTION('ref_axis',(0.,-0.499999999993262,-0.866025403788329));
#29553=DIRECTION('center_axis',(1.,0.,0.));
#29554=DIRECTION('ref_axis',(0.,0.,1.));
#29555=DIRECTION('center_axis',(-1.,0.,0.));
#29556=DIRECTION('ref_axis',(0.,0.,1.));
#29557=DIRECTION('center_axis',(1.,0.,0.));
#29558=DIRECTION('ref_axis',(0.,-0.499999999993262,0.866025403788329));
#29559=DIRECTION('center_axis',(1.,0.,0.));
#29560=DIRECTION('ref_axis',(0.,0.,1.));
#29561=DIRECTION('center_axis',(1.,0.,0.));
#29562=DIRECTION('ref_axis',(0.,-0.499999999993262,-0.866025403788329));
#29563=DIRECTION('center_axis',(1.,0.,0.));
#29564=DIRECTION('ref_axis',(0.,0.,-1.));
#29565=DIRECTION('center_axis',(-1.,0.,0.));
#29566=DIRECTION('ref_axis',(0.,-0.499999999993262,0.866025403788329));
#29567=DIRECTION('center_axis',(1.,0.,0.));
#29568=DIRECTION('ref_axis',(0.,-0.499999999993262,0.866025403788329));
#29569=DIRECTION('',(1.,0.,0.));
#29570=DIRECTION('',(-1.,0.,0.));
#29571=DIRECTION('center_axis',(-1.,0.,0.));
#29572=DIRECTION('ref_axis',(0.,1.22464679914735E-16,-1.));
#29573=DIRECTION('',(1.,0.,0.));
#29574=DIRECTION('center_axis',(1.,0.,0.));
#29575=DIRECTION('ref_axis',(0.,0.,1.));
#29576=DIRECTION('',(-1.,0.,0.));
#29577=DIRECTION('center_axis',(-1.,0.,0.));
#29578=DIRECTION('ref_axis',(0.,0.,1.));
#29579=DIRECTION('',(1.,0.,0.));
#29580=DIRECTION('center_axis',(1.,0.,0.));
#29581=DIRECTION('ref_axis',(0.,0.,1.));
#29582=DIRECTION('',(-1.,0.,0.));
#29583=DIRECTION('center_axis',(-1.,0.,0.));
#29584=DIRECTION('ref_axis',(0.,0.,1.));
#29585=DIRECTION('',(1.,0.,0.));
#29586=DIRECTION('center_axis',(1.,0.,0.));
#29587=DIRECTION('ref_axis',(0.,0.,1.));
#29588=DIRECTION('center_axis',(-1.,0.,0.));
#29589=DIRECTION('ref_axis',(0.,0.17575598334211,0.98443376329718));
#29590=DIRECTION('',(-1.,0.,0.));
#29591=DIRECTION('center_axis',(1.,0.,0.));
#29592=DIRECTION('ref_axis',(0.,-0.499999999993262,-0.866025403788329));
#29593=DIRECTION('center_axis',(-1.,0.,0.));
#29594=DIRECTION('ref_axis',(0.,-0.499999999993262,-0.866025403788329));
#29595=DIRECTION('center_axis',(1.,0.,0.));
#29596=DIRECTION('ref_axis',(0.,-0.499999999993262,-0.866025403788329));
#29597=DIRECTION('',(1.,0.,0.));
#29598=DIRECTION('center_axis',(1.,0.,0.));
#29599=DIRECTION('ref_axis',(0.,1.,0.));
#29600=DIRECTION('center_axis',(1.,0.,0.));
#29601=DIRECTION('ref_axis',(0.,0.,-1.));
#29602=DIRECTION('center_axis',(1.,0.,0.));
#29603=DIRECTION('ref_axis',(0.,1.,0.));
#29604=DIRECTION('center_axis',(1.,0.,0.));
#29605=DIRECTION('ref_axis',(0.,0.,-1.));
#29606=DIRECTION('center_axis',(1.,0.,0.));
#29607=DIRECTION('ref_axis',(0.,0.,-1.));
#29608=DIRECTION('center_axis',(1.,0.,0.));
#29609=DIRECTION('ref_axis',(0.,1.,0.));
#29610=DIRECTION('center_axis',(1.,0.,0.));
#29611=DIRECTION('ref_axis',(0.,0.,-1.));
#29612=DIRECTION('center_axis',(1.,0.,0.));
#29613=DIRECTION('ref_axis',(0.,-0.499999999993262,0.866025403788329));
#29614=DIRECTION('',(0.,0.,1.));
#29615=DIRECTION('',(0.,-1.,0.));
#29616=DIRECTION('',(0.,0.,-1.));
#29617=DIRECTION('center_axis',(1.,0.,0.));
#29618=DIRECTION('ref_axis',(0.,0.,-1.));
#29619=DIRECTION('center_axis',(-1.,0.,0.));
#29620=DIRECTION('ref_axis',(0.,-0.94042263903113,-0.340007735202781));
#29621=DIRECTION('',(-1.,0.,0.));
#29622=DIRECTION('center_axis',(-1.,0.,0.));
#29623=DIRECTION('ref_axis',(0.,1.,0.));
#29624=DIRECTION('',(1.,0.,0.));
#29625=DIRECTION('center_axis',(-1.,0.,0.));
#29626=DIRECTION('ref_axis',(0.,0.764666655685446,-0.644426028092314));
#29627=DIRECTION('',(-1.,0.,0.));
#29628=DIRECTION('center_axis',(1.,0.,0.));
#29629=DIRECTION('ref_axis',(0.,0.,-1.));
#29630=DIRECTION('',(-1.,0.,0.));
#29631=DIRECTION('',(1.,0.,0.));
#29632=DIRECTION('center_axis',(0.,0.,1.));
#29633=DIRECTION('ref_axis',(1.,0.,0.));
#29634=DIRECTION('',(-1.,0.,0.));
#29635=DIRECTION('',(1.,0.,0.));
#29636=DIRECTION('center_axis',(0.,0.,-1.));
#29637=DIRECTION('ref_axis',(-1.,0.,0.));
#29638=DIRECTION('center_axis',(0.,-1.,0.));
#29639=DIRECTION('ref_axis',(0.,0.,-1.));
#29640=DIRECTION('center_axis',(0.,1.,0.));
#29641=DIRECTION('ref_axis',(1.,0.,0.));
#29642=DIRECTION('center_axis',(0.,0.,1.));
#29643=DIRECTION('ref_axis',(-1.,0.,0.));
#29644=DIRECTION('',(0.,0.,1.));
#29645=DIRECTION('center_axis',(1.,0.,0.));
#29646=DIRECTION('ref_axis',(0.,0.,-1.));
#29647=DIRECTION('',(-1.,0.,0.));
#29648=DIRECTION('',(-1.,0.,0.));
#29649=DIRECTION('center_axis',(0.946028810149232,-0.324082536350894,7.74377105026033E-10));
#29650=DIRECTION('ref_axis',(0.0328036819517733,0.0957571728004204,-0.994864052173802));
#29651=DIRECTION('',(-1.,0.,0.));
#29652=DIRECTION('center_axis',(-0.94602881016076,0.324082536317243,7.10771293430115E-14));
#29653=DIRECTION('ref_axis',(0.0103965438556825,0.03034853443635,-0.999485306712121));
#29654=DIRECTION('',(-1.,0.,0.));
#29655=DIRECTION('center_axis',(1.,0.,0.));
#29656=DIRECTION('ref_axis',(0.,0.,-1.));
#29657=DIRECTION('',(-1.,0.,0.));
#29658=DIRECTION('center_axis',(-1.,0.,0.));
#29659=DIRECTION('ref_axis',(0.,0.,-1.));
#29660=DIRECTION('',(1.,0.,0.));
#29661=DIRECTION('center_axis',(1.,0.,0.));
#29662=DIRECTION('ref_axis',(0.,0.,-1.));
#29663=DIRECTION('',(-1.,0.,0.));
#29664=DIRECTION('center_axis',(-1.,0.,0.));
#29665=DIRECTION('ref_axis',(0.,0.,-1.));
#29666=DIRECTION('',(-1.,0.,0.));
#29667=DIRECTION('center_axis',(-1.,0.,0.));
#29668=DIRECTION('ref_axis',(0.,0.,-1.));
#29669=DIRECTION('',(1.,0.,0.));
#29670=DIRECTION('center_axis',(1.,0.,0.));
#29671=DIRECTION('ref_axis',(0.,0.,-1.));
#29672=DIRECTION('',(-1.,0.,0.));
#29673=DIRECTION('',(1.,0.,0.));
#29674=DIRECTION('center_axis',(0.50000000001139,-0.866025403777863,5.6567377117582E-14));
#29675=DIRECTION('ref_axis',(0.866025403777863,0.50000000001139,-7.49337626227376E-11));
#29676=DIRECTION('center_axis',(-0.500000000011408,-0.866025403777852,-1.85864239100662E-13));
#29677=DIRECTION('ref_axis',(0.866025403777852,-0.500000000011408,-4.16431008826601E-10));
#29678=DIRECTION('',(1.,0.,0.));
#29679=DIRECTION('center_axis',(0.500000000001134,0.866025403783784,-5.52352953831563E-15));
#29680=DIRECTION('ref_axis',(0.866025403783784,-0.500000000001134,-1.60186152837855E-11));
#29681=DIRECTION('center_axis',(-0.500000000001135,0.866025403783783,5.52352953831541E-15));
#29682=DIRECTION('ref_axis',(0.866025403783783,0.500000000001135,-3.15235664736174E-11));
#29683=DIRECTION('center_axis',(-0.855183382509445,0.518325556267202,0.));
#29684=DIRECTION('ref_axis',(0.518325556267202,0.855183382509445,0.));
#29685=DIRECTION('',(-1.,0.,0.));
#29686=DIRECTION('center_axis',(-0.855183382508501,0.518325556268759,0.));
#29687=DIRECTION('ref_axis',(0.518325556268759,0.855183382508501,0.));
#29688=DIRECTION('center_axis',(1.,0.,0.));
#29689=DIRECTION('ref_axis',(0.,0.,-1.));
#29690=DIRECTION('',(-1.,0.,0.));
#29691=DIRECTION('center_axis',(-1.,0.,0.));
#29692=DIRECTION('ref_axis',(0.,0.,-1.));
#29693=DIRECTION('',(1.,0.,0.));
#29694=DIRECTION('center_axis',(1.,0.,0.));
#29695=DIRECTION('ref_axis',(0.,0.,-1.));
#29696=DIRECTION('center_axis',(-0.829037572548639,-0.55919290348024,0.));
#29697=DIRECTION('ref_axis',(-0.55919290348024,0.829037572548639,0.));
#29698=DIRECTION('',(1.,0.,0.));
#29699=DIRECTION('center_axis',(0.82903757255312,0.559192903473596,0.));
#29700=DIRECTION('ref_axis',(-0.559192903473596,0.82903757255312,0.));
#29701=DIRECTION('center_axis',(0.500000000011392,0.866025403777861,2.42431616218218E-14));
#29702=DIRECTION('ref_axis',(0.866025403777861,-0.500000000011392,1.34504687835035E-10));
#29703=DIRECTION('',(-1.,0.,0.));
#29704=DIRECTION('center_axis',(-0.500000000001136,-0.866025403783783,8.28529430747307E-15));
#29705=DIRECTION('ref_axis',(0.866025403783783,-0.500000000001136,-3.29777777975133E-11));
#29706=DIRECTION('center_axis',(0.500000000001135,-0.866025403783783,5.5235295383155E-15));
#29707=DIRECTION('ref_axis',(0.866025403783783,0.500000000001135,-1.55386342491463E-11));
#29708=DIRECTION('',(-1.,0.,0.));
#29709=DIRECTION('center_axis',(-0.50000000001139,0.866025403777863,4.84863232436438E-14));
#29710=DIRECTION('ref_axis',(0.866025403777863,0.50000000001139,-3.46934311402352E-10));
#29711=DIRECTION('center_axis',(1.,0.,0.));
#29712=DIRECTION('ref_axis',(0.,0.,-1.));
#29713=DIRECTION('center_axis',(-1.,0.,0.));
#29714=DIRECTION('ref_axis',(0.,0.,-1.));
#29715=DIRECTION('',(1.,0.,0.));
#29716=DIRECTION('center_axis',(-1.,0.,0.));
#29717=DIRECTION('ref_axis',(0.,0.,-1.));
#29718=DIRECTION('',(-1.,0.,0.));
#29719=DIRECTION('center_axis',(1.,0.,0.));
#29720=DIRECTION('ref_axis',(0.,0.,-1.));
#29721=DIRECTION('',(1.,0.,0.));
#29722=DIRECTION('center_axis',(1.,0.,0.));
#29723=DIRECTION('ref_axis',(0.,0.,-1.));
#29724=DIRECTION('',(1.,0.,0.));
#29725=DIRECTION('center_axis',(-1.,0.,0.));
#29726=DIRECTION('ref_axis',(0.,0.,1.));
#29727=DIRECTION('',(0.,0.,-1.));
#29728=DIRECTION('',(0.,0.,-1.));
#29729=DIRECTION('center_axis',(0.,1.,0.));
#29730=DIRECTION('ref_axis',(1.,0.,0.));
#29731=DIRECTION('',(0.,0.,-1.));
#29732=DIRECTION('center_axis',(0.,1.,0.));
#29733=DIRECTION('ref_axis',(1.,0.,0.));
#29734=DIRECTION('',(0.,0.,-1.));
#29735=DIRECTION('center_axis',(-1.,0.,0.));
#29736=DIRECTION('ref_axis',(0.,0.,1.));
#29737=DIRECTION('',(0.,0.,-1.));
#29738=DIRECTION('center_axis',(0.,-1.,0.));
#29739=DIRECTION('ref_axis',(0.,0.,-1.));
#29740=DIRECTION('',(0.,0.,-1.));
#29741=DIRECTION('center_axis',(1.,0.,0.));
#29742=DIRECTION('ref_axis',(0.,1.,0.));
#29743=DIRECTION('',(0.,0.,-1.));
#29744=DIRECTION('center_axis',(0.,1.,0.));
#29745=DIRECTION('ref_axis',(1.,0.,0.));
#29746=DIRECTION('',(0.,0.,-1.));
#29747=DIRECTION('center_axis',(1.,0.,0.));
#29748=DIRECTION('ref_axis',(0.,1.,0.));
#29749=DIRECTION('center_axis',(-0.855183382508501,0.518325556268759,0.));
#29750=DIRECTION('ref_axis',(0.,0.,1.));
#29751=DIRECTION('',(0.,0.,-1.));
#29752=DIRECTION('center_axis',(0.855183382508501,-0.518325556268759,0.));
#29753=DIRECTION('ref_axis',(0.518325556268759,0.855183382508501,0.));
#29754=DIRECTION('',(0.,0.,-1.));
#29755=DIRECTION('center_axis',(0.,1.,0.));
#29756=DIRECTION('ref_axis',(1.,0.,0.));
#29757=DIRECTION('',(0.,0.,-1.));
#29758=DIRECTION('',(1.,0.,0.));
#29759=DIRECTION('center_axis',(0.855183382509445,-0.518325556267202,0.));
#29760=DIRECTION('ref_axis',(0.,0.,-1.));
#29761=DIRECTION('',(0.,0.,-1.));
#29762=DIRECTION('center_axis',(0.855183382509445,-0.518325556267202,0.));
#29763=DIRECTION('ref_axis',(0.518325556267202,0.855183382509445,0.));
#29764=DIRECTION('center_axis',(0.,-1.,0.));
#29765=DIRECTION('ref_axis',(0.,0.,-1.));
#29766=DIRECTION('',(0.,0.,-1.));
#29767=DIRECTION('',(-1.,0.,0.));
#29768=DIRECTION('',(0.,0.,-1.));
#29769=DIRECTION('center_axis',(-0.829037572548639,-0.55919290348024,0.));
#29770=DIRECTION('ref_axis',(-0.55919290348024,0.829037572548639,0.));
#29771=DIRECTION('',(0.,0.,-1.));
#29772=DIRECTION('center_axis',(0.829037572548639,0.55919290348024,0.));
#29773=DIRECTION('ref_axis',(-0.55919290348024,0.829037572548639,0.));
#29774=DIRECTION('center_axis',(1.,0.,0.));
#29775=DIRECTION('ref_axis',(0.,1.,0.));
#29776=DIRECTION('',(0.,0.,-1.));
#29777=DIRECTION('center_axis',(-1.,0.,0.));
#29778=DIRECTION('ref_axis',(0.,0.,-1.));
#29779=DIRECTION('center_axis',(0.,-1.,0.));
#29780=DIRECTION('ref_axis',(0.,0.,-1.));
#29781=DIRECTION('',(0.,0.,-1.));
#29782=DIRECTION('',(-1.,0.,0.));
#29783=DIRECTION('center_axis',(-1.,0.,0.));
#29784=DIRECTION('ref_axis',(0.,0.,1.));
#29785=DIRECTION('',(0.,0.,-1.));
#29786=DIRECTION('center_axis',(1.,0.,0.));
#29787=DIRECTION('ref_axis',(0.,0.,-1.));
#29788=DIRECTION('center_axis',(0.,1.,0.));
#29789=DIRECTION('ref_axis',(1.,0.,0.));
#29790=DIRECTION('',(0.,0.,-1.));
#29791=DIRECTION('',(1.,0.,0.));
#29792=DIRECTION('center_axis',(1.,0.,0.));
#29793=DIRECTION('ref_axis',(0.,1.,0.));
#29794=DIRECTION('center_axis',(-1.,0.,0.));
#29795=DIRECTION('ref_axis',(0.,0.,-1.));
#29796=DIRECTION('center_axis',(0.82903757255312,0.559192903473596,0.));
#29797=DIRECTION('ref_axis',(0.,0.,-1.));
#29798=DIRECTION('center_axis',(-0.82903757255312,-0.559192903473596,0.));
#29799=DIRECTION('ref_axis',(-0.559192903473596,0.82903757255312,0.));
#29800=DIRECTION('center_axis',(1.,0.,0.));
#29801=DIRECTION('ref_axis',(0.,0.,-1.));
#29802=DIRECTION('center_axis',(1.,0.,0.));
#29803=DIRECTION('ref_axis',(0.,0.,-1.));
#29804=DIRECTION('center_axis',(-0.500000000001133,-0.866025403783785,1.87875446695563E-14));
#29805=DIRECTION('ref_axis',(0.866025403783785,-0.500000000001133,1.73760906682291E-11));
#29806=DIRECTION('',(-1.,0.,0.));
#29807=DIRECTION('center_axis',(0.500000000011412,0.86602540377785,2.35812383115421E-13));
#29808=DIRECTION('ref_axis',(0.86602540377785,-0.500000000011412,4.13106356090107E-10));
#29809=DIRECTION('center_axis',(-0.500000000011409,0.866025403777852,1.88649906492394E-13));
#29810=DIRECTION('ref_axis',(0.866025403777852,0.500000000011409,-1.71455444984074E-12));
#29811=DIRECTION('',(-1.,0.,0.));
#29812=DIRECTION('center_axis',(0.500000000001134,-0.866025403783784,2.6839349527939E-15));
#29813=DIRECTION('ref_axis',(0.866025403783784,0.500000000001134,2.2215382786634E-11));
#29814=DIRECTION('center_axis',(-0.500000000011394,-0.866025403777861,0.));
#29815=DIRECTION('ref_axis',(-0.866025403777861,0.500000000011394,0.));
#29816=DIRECTION('',(0.,0.,-1.));
#29817=DIRECTION('',(0.,0.,-1.));
#29818=DIRECTION('center_axis',(0.500000000011394,-0.866025403777861,0.));
#29819=DIRECTION('ref_axis',(0.,0.,-1.));
#29820=DIRECTION('',(0.,0.,-1.));
#29821=DIRECTION('center_axis',(0.,-1.,0.));
#29822=DIRECTION('ref_axis',(0.,0.,-1.));
#29823=DIRECTION('',(0.,0.,-1.));
#29824=DIRECTION('center_axis',(0.500000000001135,0.866025403783784,0.));
#29825=DIRECTION('ref_axis',(0.,0.,-1.));
#29826=DIRECTION('',(0.,0.,-1.));
#29827=DIRECTION('center_axis',(-0.500000000001135,0.866025403783784,0.));
#29828=DIRECTION('ref_axis',(0.,0.,1.));
#29829=DIRECTION('',(0.,0.,-1.));
#29830=DIRECTION('center_axis',(0.,-1.,0.));
#29831=DIRECTION('ref_axis',(0.,0.,-1.));
#29832=DIRECTION('center_axis',(0.,1.,0.));
#29833=DIRECTION('ref_axis',(1.,0.,0.));
#29834=DIRECTION('',(0.,0.,-1.));
#29835=DIRECTION('',(1.,0.,0.));
#29836=DIRECTION('',(0.,0.,-1.));
#29837=DIRECTION('center_axis',(0.500000000001135,-0.866025403783784,0.));
#29838=DIRECTION('ref_axis',(0.,0.,-1.));
#29839=DIRECTION('',(0.,0.,-1.));
#29840=DIRECTION('center_axis',(-0.500000000001134,0.866025403783784,1.34196747639693E-14));
#29841=DIRECTION('ref_axis',(0.866025403783784,0.500000000001134,-2.93336016297228E-11));
#29842=DIRECTION('center_axis',(-0.500000000001135,-0.866025403783784,0.));
#29843=DIRECTION('ref_axis',(-0.866025403783784,0.500000000001135,0.));
#29844=DIRECTION('',(0.,0.,-1.));
#29845=DIRECTION('center_axis',(0.500000000001132,0.866025403783785,2.41554145751436E-14));
#29846=DIRECTION('ref_axis',(0.866025403783785,-0.500000000001132,1.58006467766065E-11));
#29847=DIRECTION('center_axis',(0.,1.,0.));
#29848=DIRECTION('ref_axis',(1.,0.,0.));
#29849=DIRECTION('',(0.,0.,-1.));
#29850=DIRECTION('',(1.,0.,0.));
#29851=DIRECTION('center_axis',(-0.500000000011394,0.866025403777861,0.));
#29852=DIRECTION('ref_axis',(0.,0.,1.));
#29853=DIRECTION('center_axis',(0.500000000011412,-0.86602540377785,2.35812383115473E-13));
#29854=DIRECTION('ref_axis',(0.86602540377785,0.500000000011412,1.59264985720823E-10));
#29855=DIRECTION('',(0.,0.,-1.));
#29856=DIRECTION('center_axis',(0.500000000011394,0.866025403777861,0.));
#29857=DIRECTION('ref_axis',(0.,0.,-1.));
#29858=DIRECTION('center_axis',(-0.500000000011402,-0.866025403777856,1.17906191557739E-13));
#29859=DIRECTION('ref_axis',(0.866025403777856,-0.500000000011402,-2.60506588040655E-10));
#29860=DIRECTION('center_axis',(1.,0.,0.));
#29861=DIRECTION('ref_axis',(0.,0.,-1.));
#29862=DIRECTION('center_axis',(-0.946028810160758,0.324082536317247,0.));
#29863=DIRECTION('ref_axis',(0.,0.,1.));
#29864=DIRECTION('',(0.,0.,-1.));
#29865=DIRECTION('center_axis',(0.94602881016076,-0.324082536317242,-7.53842350672448E-14));
#29866=DIRECTION('ref_axis',(0.033646559749939,0.0982176184129628,-0.99459600263136));
#29867=DIRECTION('',(0.,0.,-1.));
#29868=DIRECTION('center_axis',(0.,1.,0.));
#29869=DIRECTION('ref_axis',(1.,0.,0.));
#29870=DIRECTION('',(0.,0.,-1.));
#29871=DIRECTION('',(1.,0.,0.));
#29872=DIRECTION('center_axis',(0.946028810171404,-0.324082536286173,0.));
#29873=DIRECTION('ref_axis',(0.,0.,-1.));
#29874=DIRECTION('',(0.,0.,-1.));
#29875=DIRECTION('center_axis',(-0.946028810149238,0.324082536350876,-7.54583899480575E-10));
#29876=DIRECTION('ref_axis',(0.00721450072149016,0.0210598351143057,-0.999752186456373));
#29877=DIRECTION('center_axis',(0.,0.,-1.));
#29878=DIRECTION('ref_axis',(0.587785252292473,0.809016994374947,0.));
#29879=DIRECTION('',(0.,0.,-1.));
#29880=DIRECTION('center_axis',(0.,-1.,0.));
#29881=DIRECTION('ref_axis',(0.,0.,-1.));
#29882=DIRECTION('',(0.,0.,-1.));
#29883=DIRECTION('',(-1.,0.,0.));
#29884=DIRECTION('center_axis',(-1.,0.,0.));
#29885=DIRECTION('ref_axis',(0.,0.,1.));
#29886=DIRECTION('',(0.,0.,-1.));
#29887=DIRECTION('center_axis',(-1.,0.,0.));
#29888=DIRECTION('ref_axis',(0.,0.,-1.));
#29889=DIRECTION('',(0.,0.,-1.));
#29890=DIRECTION('center_axis',(0.,-1.,0.));
#29891=DIRECTION('ref_axis',(0.,0.,-1.));
#29892=DIRECTION('',(0.,0.,-1.));
#29893=DIRECTION('',(1.,0.,0.));
#29894=DIRECTION('center_axis',(-1.,0.,0.));
#29895=DIRECTION('ref_axis',(0.,0.,1.));
#29896=DIRECTION('',(0.,0.,-1.));
#29897=DIRECTION('center_axis',(1.,0.,0.));
#29898=DIRECTION('ref_axis',(0.,0.,-1.));
#29899=DIRECTION('center_axis',(0.,1.,0.));
#29900=DIRECTION('ref_axis',(1.,0.,0.));
#29901=DIRECTION('',(0.,0.,-1.));
#29902=DIRECTION('',(1.,0.,0.));
#29903=DIRECTION('center_axis',(1.,0.,0.));
#29904=DIRECTION('ref_axis',(0.,1.,0.));
#29905=DIRECTION('',(0.,0.,-1.));
#29906=DIRECTION('center_axis',(-1.,0.,0.));
#29907=DIRECTION('ref_axis',(0.,0.,-1.));
#29908=DIRECTION('center_axis',(0.,1.,0.));
#29909=DIRECTION('ref_axis',(1.,0.,0.));
#29910=DIRECTION('',(1.,0.,0.));
#29911=DIRECTION('center_axis',(0.,0.,-1.));
#29912=DIRECTION('ref_axis',(0.,1.,0.));
#29913=DIRECTION('',(0.,0.,-1.));
#29914=DIRECTION('center_axis',(0.,1.,0.));
#29915=DIRECTION('ref_axis',(1.,0.,0.));
#29916=DIRECTION('',(-1.,0.,0.));
#29917=DIRECTION('center_axis',(1.,0.,0.));
#29918=DIRECTION('ref_axis',(0.,0.,-1.));
#51705=CARTESIAN_POINT('',(0.,0.,0.));
#51706=CARTESIAN_POINT('Origin',(-6.,0.,-10.));
#51707=CARTESIAN_POINT('',(-6.,-11.5470739757602,3.26574380475891));
#51708=CARTESIAN_POINT('',(-6.,-19.921468401738,1.77062043322529));
#51709=CARTESIAN_POINT('Origin',(-6.,-13.8564064606,-8.));
#51710=CARTESIAN_POINT('',(-6.,-11.4941364764755,16.3671875));
#51711=CARTESIAN_POINT('Origin',(-6.,0.,0.));
#51712=CARTESIAN_POINT('',(-6.,-8.60175408505985,8.3671875));
#51713=CARTESIAN_POINT('Origin',(-6.,0.,16.));
#51714=CARTESIAN_POINT('Origin',(-6.,0.,0.));
#51715=CARTESIAN_POINT('Origin',(33.,0.,-9.5));
#51716=CARTESIAN_POINT('',(33.,2.32682891837997E-15,19.));
#51717=CARTESIAN_POINT('Origin',(33.,0.,0.));
#51718=CARTESIAN_POINT('',(33.,2.5,9.3));
#51719=CARTESIAN_POINT('',(33.,2.5,6.53834841531101));
#51720=CARTESIAN_POINT('',(33.,2.5,-2.425));
#51721=CARTESIAN_POINT('',(33.,-2.5,6.53834841531101));
#51722=CARTESIAN_POINT('Origin',(33.,0.,0.));
#51723=CARTESIAN_POINT('',(33.,-2.5,9.3));
#51724=CARTESIAN_POINT('',(33.,-2.5,-2.425));
#51725=CARTESIAN_POINT('',(33.,0.,9.3));
#51726=CARTESIAN_POINT('Origin',(32.5,0.,0.));
#51727=CARTESIAN_POINT('',(32.,2.44929359829471E-15,20.));
#51728=CARTESIAN_POINT('Origin',(32.,0.,0.));
#51729=CARTESIAN_POINT('',(32.5,2.38806125833734E-15,19.5));
#51730=CARTESIAN_POINT('Origin',(13.,0.,0.));
#51731=CARTESIAN_POINT('',(3.7202200813,-0.2994444445,-19.9977581999748));
#51732=CARTESIAN_POINT('',(4.3435534146,-0.2994444445,-19.9977581999748));
#51733=CARTESIAN_POINT('',(4.03188674795,-0.2994444445,-19.9977581999748));
#51734=CARTESIAN_POINT('',(4.3435534146,-1.1061111111,-19.969389530226));
#51735=CARTESIAN_POINT('Ctrl Pts',(4.3435534146,-0.2994444445,-19.9977581999748));
#51736=CARTESIAN_POINT('Ctrl Pts',(4.39419529583398,-0.2994444445,-19.9977581999748));
#51737=CARTESIAN_POINT('Ctrl Pts',(4.44821240138141,-0.309565031449933,
-19.9976146851541));
#51738=CARTESIAN_POINT('Ctrl Pts',(4.54758041279513,-0.350722737591021,
-19.9969351943239));
#51739=CARTESIAN_POINT('Ctrl Pts',(4.59293124895252,-0.381759842781414,
-19.9963882206146));
#51740=CARTESIAN_POINT('Ctrl Pts',(4.66456114163788,-0.453382333903515,
-19.994892548385));
#51741=CARTESIAN_POINT('Ctrl Pts',(4.69560697302298,-0.498746314496724,
-19.993842130762));
#51742=CARTESIAN_POINT('Ctrl Pts',(4.73676959169473,-0.5981279615852,-19.9911158762495));
#51743=CARTESIAN_POINT('Ctrl Pts',(4.7468867479,-0.652145173345914,-19.9894290439444));
#51744=CARTESIAN_POINT('Ctrl Pts',(4.7468867479,-0.753438288963382,-19.9858675169476));
#51745=CARTESIAN_POINT('Ctrl Pts',(4.73675961734101,-0.80746838265751,-19.9837551246746));
#51746=CARTESIAN_POINT('Ctrl Pts',(4.69558023913546,-0.906857064706403,
-19.9794915935354));
#51747=CARTESIAN_POINT('Ctrl Pts',(4.66452814741898,-0.952216188266304,
-19.9773514320566));
#51748=CARTESIAN_POINT('Ctrl Pts',(4.59290252845076,-1.02381445280548,-19.9738100392531));
#51749=CARTESIAN_POINT('Ctrl Pts',(4.54756443095206,-1.05484068319396,-19.9721740344373));
#51750=CARTESIAN_POINT('Ctrl Pts',(4.44821243395584,-1.09598926486806,-19.9699582388217));
#51751=CARTESIAN_POINT('Ctrl Pts',(4.39419807843,-1.1061111111,-19.969389530226));
#51752=CARTESIAN_POINT('Ctrl Pts',(4.3435534146,-1.1061111111,-19.969389530226));
#51753=CARTESIAN_POINT('',(3.7202200813,-1.1061111111,-19.969389530226));
#51754=CARTESIAN_POINT('',(4.03188674795,-1.1061111111,-19.969389530226));
#51755=CARTESIAN_POINT('Origin',(3.7202200813,0.,0.));
#51756=CARTESIAN_POINT('Origin',(-6.,0.,-10.));
#51757=CARTESIAN_POINT('',(-6.,8.60175408505985,8.3671875));
#51758=CARTESIAN_POINT('',(-6.,11.4941364764755,16.3671875));
#51759=CARTESIAN_POINT('Origin',(-6.,0.,16.));
#51760=CARTESIAN_POINT('',(-6.,19.921468401738,1.77062043322529));
#51761=CARTESIAN_POINT('Origin',(-6.,0.,0.));
#51762=CARTESIAN_POINT('',(-6.,11.5470739757602,3.26574380475891));
#51763=CARTESIAN_POINT('Origin',(-6.,13.8564064606,-8.));
#51764=CARTESIAN_POINT('Origin',(-6.,0.,0.));
#51765=CARTESIAN_POINT('Origin',(-6.,0.,-10.));
#51766=CARTESIAN_POINT('',(-6.,-8.42733192529161,-18.1378079331809));
#51767=CARTESIAN_POINT('',(-6.,-2.94531989074286,-11.632931304757));
#51768=CARTESIAN_POINT('Origin',(-6.,-13.8564064606,-8.));
#51769=CARTESIAN_POINT('',(-6.,2.94531989074286,-11.632931304757));
#51770=CARTESIAN_POINT('Origin',(-6.,0.,0.));
#51771=CARTESIAN_POINT('',(-6.,8.42733192529161,-18.1378079331809));
#51772=CARTESIAN_POINT('Origin',(-6.,13.8564064606,-8.));
#51773=CARTESIAN_POINT('Origin',(-6.,0.,0.));
#51774=CARTESIAN_POINT('Origin',(1.,-13.8564064606,-8.));
#51775=CARTESIAN_POINT('',(8.,-11.5470739757602,3.26574380475891));
#51776=CARTESIAN_POINT('',(8.,-19.921468401738,1.77062043322529));
#51777=CARTESIAN_POINT('Origin',(8.,-13.8564064606,-8.));
#51778=CARTESIAN_POINT('',(1.,-19.921468401738,1.77062043322529));
#51779=CARTESIAN_POINT('',(1.,-11.5470739757602,3.26574380475891));
#51780=CARTESIAN_POINT('Origin',(1.,0.,0.));
#51781=CARTESIAN_POINT('',(8.,-2.94531989074286,-11.632931304757));
#51782=CARTESIAN_POINT('',(1.,-2.94531989074286,-11.632931304757));
#51783=CARTESIAN_POINT('',(8.,2.94531989074286,-11.632931304757));
#51784=CARTESIAN_POINT('Origin',(8.,0.,0.));
#51785=CARTESIAN_POINT('',(1.,2.94531989074286,-11.632931304757));
#51786=CARTESIAN_POINT('Origin',(1.,0.,0.));
#51787=CARTESIAN_POINT('',(8.,11.5470739757602,3.26574380475891));
#51788=CARTESIAN_POINT('',(1.,11.5470739757602,3.26574380475891));
#51789=CARTESIAN_POINT('',(8.,8.60175408505985,8.3671875));
#51790=CARTESIAN_POINT('Origin',(8.,0.,0.));
#51791=CARTESIAN_POINT('',(1.,8.60175408505985,8.3671875));
#51792=CARTESIAN_POINT('Origin',(1.,0.,0.));
#51793=CARTESIAN_POINT('',(8.,-8.60175408505985,8.3671875));
#51794=CARTESIAN_POINT('',(1.,-8.60175408505985,8.3671875));
#51795=CARTESIAN_POINT('Origin',(8.,0.,0.));
#51796=CARTESIAN_POINT('Origin',(1.,13.8564064606,-8.));
#51797=CARTESIAN_POINT('',(8.,19.921468401738,1.77062043322529));
#51798=CARTESIAN_POINT('',(1.,19.921468401738,1.77062043322529));
#51799=CARTESIAN_POINT('Origin',(8.,13.8564064606,-8.));
#51800=CARTESIAN_POINT('Origin',(1.,13.8564064606,-8.));
#51801=CARTESIAN_POINT('',(8.,8.42733192529161,-18.1378079331809));
#51802=CARTESIAN_POINT('Origin',(8.,13.8564064606,-8.));
#51803=CARTESIAN_POINT('',(1.,8.42733192529161,-18.1378079331809));
#51804=CARTESIAN_POINT('Origin',(8.,13.8564064606,-8.));
#51805=CARTESIAN_POINT('',(8.,-8.42733192529161,-18.1378079331809));
#51806=CARTESIAN_POINT('Origin',(8.,0.,0.));
#51807=CARTESIAN_POINT('',(8.,-11.4941364764755,16.3671875));
#51808=CARTESIAN_POINT('Origin',(8.,0.,16.));
#51809=CARTESIAN_POINT('',(8.,-2.44929359829471E-15,20.));
#51810=CARTESIAN_POINT('Origin',(8.,0.,0.));
#51811=CARTESIAN_POINT('',(8.,11.4941364764755,16.3671875));
#51812=CARTESIAN_POINT('Origin',(8.,0.,0.));
#51813=CARTESIAN_POINT('Origin',(8.,0.,16.));
#51814=CARTESIAN_POINT('Origin',(8.,0.,0.));
#51815=CARTESIAN_POINT('Origin',(8.,-13.8564064606,-8.));
#51816=CARTESIAN_POINT('',(8.,2.5,6.53834841531101));
#51817=CARTESIAN_POINT('',(8.,2.5,9.3));
#51818=CARTESIAN_POINT('',(8.,2.5,-1.675));
#51819=CARTESIAN_POINT('',(8.,-2.5,9.3));
#51820=CARTESIAN_POINT('',(8.,6.9282032303,9.3));
#51821=CARTESIAN_POINT('',(8.,-2.5,6.53834841531101));
#51822=CARTESIAN_POINT('',(8.,-2.5,-1.675));
#51823=CARTESIAN_POINT('Origin',(8.,0.,0.));
#51824=CARTESIAN_POINT('Origin',(1.,0.,16.));
#51825=CARTESIAN_POINT('',(1.,-11.4941364764755,16.3671875));
#51826=CARTESIAN_POINT('Origin',(1.,0.,16.));
#51827=CARTESIAN_POINT('',(1.,11.4941364764755,16.3671875));
#51828=CARTESIAN_POINT('Origin',(1.,-13.8564064606,-8.));
#51829=CARTESIAN_POINT('',(1.,-8.42733192529161,-18.1378079331809));
#51830=CARTESIAN_POINT('Origin',(20.5,0.,0.));
#51831=CARTESIAN_POINT('',(20.5,-2.5,6.53834841531101));
#51832=CARTESIAN_POINT('',(20.5,2.5,6.53834841531101));
#51833=CARTESIAN_POINT('Origin',(20.5,0.,9.3));
#51834=CARTESIAN_POINT('',(20.5,2.5,9.3));
#51835=CARTESIAN_POINT('',(20.5,-2.5,9.3));
#51836=CARTESIAN_POINT('',(25.1,-2.57175827820944E-16,9.3));
#51837=CARTESIAN_POINT('Origin',(23.,0.,9.3));
#51838=CARTESIAN_POINT('Origin',(20.5,2.5,4.65));
#51839=CARTESIAN_POINT('Origin',(20.5,-2.5,4.65));
#51840=CARTESIAN_POINT('Origin',(23.,0.,10.));
#51841=CARTESIAN_POINT('',(25.1,2.57175827820944E-16,20.));
#51842=CARTESIAN_POINT('',(25.1,2.57175827820944E-16,10.));
#51843=CARTESIAN_POINT('',(20.9,0.,20.));
#51844=CARTESIAN_POINT('Ctrl Pts',(20.9,4.16333634234434E-16,20.));
#51845=CARTESIAN_POINT('Ctrl Pts',(20.9,0.263888990751172,20.));
#51846=CARTESIAN_POINT('Ctrl Pts',(20.9527780741314,0.545235237847868,19.9942425936951));
#51847=CARTESIAN_POINT('Ctrl Pts',(21.1671514943451,1.06257490219278,19.97343117591));
#51848=CARTESIAN_POINT('Ctrl Pts',(21.3287361087815,1.29858458976497,19.9586721250997));
#51849=CARTESIAN_POINT('Ctrl Pts',(21.7014161819223,1.67126466290584,19.9309254589373));
#51850=CARTESIAN_POINT('Ctrl Pts',(21.9374255317885,1.83284867450471,19.9161307432363));
#51851=CARTESIAN_POINT('Ctrl Pts',(22.4547640622183,2.04722164681422,19.8952376620524));
#51852=CARTESIAN_POINT('Ctrl Pts',(22.7361099164069,2.1,19.8894444366855));
#51853=CARTESIAN_POINT('Ctrl Pts',(23.2638900835931,2.1,19.8894444366855));
#51854=CARTESIAN_POINT('Ctrl Pts',(23.5452359377817,2.04722164681422,19.8952376620524));
#51855=CARTESIAN_POINT('Ctrl Pts',(24.0625744682115,1.83284867450471,19.9161307432363));
#51856=CARTESIAN_POINT('Ctrl Pts',(24.2985838180777,1.67126466290584,19.9309254589373));
#51857=CARTESIAN_POINT('Ctrl Pts',(24.6712638912185,1.29858458976497,19.9586721250997));
#51858=CARTESIAN_POINT('Ctrl Pts',(24.8328485056549,1.06257490219277,19.97343117591));
#51859=CARTESIAN_POINT('Ctrl Pts',(25.0472219258686,0.545235237847867,19.9942425936951));
#51860=CARTESIAN_POINT('Ctrl Pts',(25.1,0.263888990751172,20.));
#51861=CARTESIAN_POINT('Ctrl Pts',(25.1,-6.93889390390723E-17,20.));
#51862=CARTESIAN_POINT('',(23.,-2.1,19.8894444366855));
#51863=CARTESIAN_POINT('Ctrl Pts',(23.,-2.1,19.8894444366855));
#51864=CARTESIAN_POINT('Ctrl Pts',(22.7361099164069,-2.1,19.8894444366855));
#51865=CARTESIAN_POINT('Ctrl Pts',(22.4547640622183,-2.04722164681422,19.8952376620524));
#51866=CARTESIAN_POINT('Ctrl Pts',(21.9374255317885,-1.83284867450471,19.9161307432363));
#51867=CARTESIAN_POINT('Ctrl Pts',(21.7014161819223,-1.67126466290584,19.9309254589373));
#51868=CARTESIAN_POINT('Ctrl Pts',(21.3287361087815,-1.29858458976497,19.9586721250997));
#51869=CARTESIAN_POINT('Ctrl Pts',(21.1671514943451,-1.06257490219277,19.97343117591));
#51870=CARTESIAN_POINT('Ctrl Pts',(20.9527780741314,-0.545235237847867,
19.9942425936951));
#51871=CARTESIAN_POINT('Ctrl Pts',(20.9,-0.263888990751171,20.));
#51872=CARTESIAN_POINT('Ctrl Pts',(20.9,-5.20417042793042E-17,20.));
#51873=CARTESIAN_POINT('Ctrl Pts',(25.1,-3.46944695195361E-16,20.));
#51874=CARTESIAN_POINT('Ctrl Pts',(25.1,-0.263888990751172,20.));
#51875=CARTESIAN_POINT('Ctrl Pts',(25.0472219258686,-0.545235237847867,
19.9942425936951));
#51876=CARTESIAN_POINT('Ctrl Pts',(24.8328485056549,-1.06257490219277,19.97343117591));
#51877=CARTESIAN_POINT('Ctrl Pts',(24.6712638912185,-1.29858458976497,19.9586721250997));
#51878=CARTESIAN_POINT('Ctrl Pts',(24.2985838180777,-1.67126466290584,19.9309254589373));
#51879=CARTESIAN_POINT('Ctrl Pts',(24.0625744682115,-1.83284867450471,19.9161307432363));
#51880=CARTESIAN_POINT('Ctrl Pts',(23.5452359377817,-2.04722164681422,19.8952376620524));
#51881=CARTESIAN_POINT('Ctrl Pts',(23.2638900835931,-2.1,19.8894444366855));
#51882=CARTESIAN_POINT('Ctrl Pts',(23.,-2.1,19.8894444366855));
#51883=CARTESIAN_POINT('Origin',(13.,0.,0.));
#51884=CARTESIAN_POINT('',(13.,-2.44929359829471E-15,20.));
#51885=CARTESIAN_POINT('',(13.,-2.44929359829471E-15,20.));
#51886=CARTESIAN_POINT('',(4.3435534146,-2.1388888889,-19.8852999555184));
#51887=CARTESIAN_POINT('',(5.18767834635794,0.459060516890588,-19.9947308919583));
#51888=CARTESIAN_POINT('Ctrl Pts',(5.18767834635794,0.459060516890587,-19.9947308919583));
#51889=CARTESIAN_POINT('Ctrl Pts',(5.24968129137097,0.414012740477042,-19.9957651472147));
#51890=CARTESIAN_POINT('Ctrl Pts',(5.30716488138641,0.364591710747686,-19.9967442102515));
#51891=CARTESIAN_POINT('Ctrl Pts',(5.48665323742873,0.185057927007366,-19.9995504652193));
#51892=CARTESIAN_POINT('Ctrl Pts',(5.59715741138799,0.0235509943668747,
-20.0007685496482));
#51893=CARTESIAN_POINT('Ctrl Pts',(5.7436627884403,-0.330259044510279,-19.9980555602176));
#51894=CARTESIAN_POINT('Ctrl Pts',(5.7796645257,-0.522560848653025,-19.993985306904));
#51895=CARTESIAN_POINT('Ctrl Pts',(5.7796645257,-0.883349185014401,-19.9812997715422));
#51896=CARTESIAN_POINT('Ctrl Pts',(5.74353603624199,-1.07581469312434,-19.971831595325));
#51897=CARTESIAN_POINT('Ctrl Pts',(5.59681775573534,-1.4297140658822,-19.9496203526915));
#51898=CARTESIAN_POINT('Ctrl Pts',(5.48623409908571,-1.59115913013439,-19.9370154287515));
#51899=CARTESIAN_POINT('Ctrl Pts',(5.23128841814184,-1.84591622773468,-19.9150423979699));
#51900=CARTESIAN_POINT('Ctrl Pts',(5.06995436664432,-1.95632911293912,-19.9042256075891));
#51901=CARTESIAN_POINT('Ctrl Pts',(4.71629161866783,-2.10281902804406,-19.8892828626319));
#51902=CARTESIAN_POINT('Ctrl Pts',(4.52395392331701,-2.1388888889,-19.8852999555184));
#51903=CARTESIAN_POINT('Ctrl Pts',(4.3435534146,-2.1388888889,-19.8852999555184));
#51904=CARTESIAN_POINT('',(5.7631397208,2.1388888889,-19.8852999555184));
#51905=CARTESIAN_POINT('Origin',(5.03059422324816,0.0005165593435702,2.33120559308216));
#51906=CARTESIAN_POINT('',(4.7295794663,2.1388888889,-19.8852999555184));
#51907=CARTESIAN_POINT('',(5.24635959355,2.1388888889,-19.8852999555184));
#51908=CARTESIAN_POINT('',(4.2292347159,0.6783333333,-19.9884932871123));
#51909=CARTESIAN_POINT('Origin',(3.99709194624176,0.000685748014040422,
2.32885472330861));
#51910=CARTESIAN_POINT('',(3.7202200813,0.6783333333,-19.9884932871123));
#51911=CARTESIAN_POINT('',(3.9747273986,0.6783333333,-19.9884932871123));
#51912=CARTESIAN_POINT('',(3.7202200813,2.1388888889,-19.8852999555184));
#51913=CARTESIAN_POINT('Origin',(3.7202200813,0.,0.));
#51914=CARTESIAN_POINT('',(2.7424423035,2.1388888889,-19.8852999555184));
#51915=CARTESIAN_POINT('',(3.2313311924,2.1388888889,-19.8852999555184));
#51916=CARTESIAN_POINT('',(2.7424423035,-2.1388888889,-19.8852999555184));
#51917=CARTESIAN_POINT('Origin',(2.7424423035,0.,0.));
#51918=CARTESIAN_POINT('',(3.54299785905,-2.1388888889,-19.8852999555184));
#51919=CARTESIAN_POINT('',(1.4888888889,-1.1611111111,-19.9662670769395));
#51920=CARTESIAN_POINT('',(1.4888888889,2.1388888889,-19.8852999555184));
#51921=CARTESIAN_POINT('Origin',(1.4888888889,0.,0.));
#51922=CARTESIAN_POINT('',(0.5111111111,2.1388888889,-19.8852999555184));
#51923=CARTESIAN_POINT('',(1.,2.1388888889,-19.8852999555184));
#51924=CARTESIAN_POINT('',(0.5111111111,-1.1611111111,-19.9662670769395));
#51925=CARTESIAN_POINT('Origin',(0.5111111111,0.,0.));
#51926=CARTESIAN_POINT('',(-0.5277777778,-1.1611111111,-19.9662670769395));
#51927=CARTESIAN_POINT('',(-0.00833333335000042,-1.1611111111,-19.9662670769395));
#51928=CARTESIAN_POINT('',(-0.5277777778,-2.1388888889,-19.8852999555184));
#51929=CARTESIAN_POINT('Origin',(-0.527777777800001,0.,0.));
#51930=CARTESIAN_POINT('',(2.5277777778,-2.1388888889,-19.8852999555184));
#51931=CARTESIAN_POINT('',(1.,-2.1388888889,-19.8852999555184));
#51932=CARTESIAN_POINT('',(2.5277777778,-1.1611111111,-19.9662670769395));
#51933=CARTESIAN_POINT('Origin',(2.5277777778,0.,0.));
#51934=CARTESIAN_POINT('',(2.00833333335,-1.1611111111,-19.9662670769395));
#51935=CARTESIAN_POINT('',(-3.7631397208,2.75,-19.8100353356575));
#51936=CARTESIAN_POINT('',(-1.8075841652,2.75,-19.8100353356575));
#51937=CARTESIAN_POINT('',(-2.785361943,2.75,-19.8100353356575));
#51938=CARTESIAN_POINT('',(1.,4.3709594736,-19.5165241085637));
#51939=CARTESIAN_POINT('Origin',(-6.57072388981035,-2.27381335982102E-9,
1.34364674941878E-8));
#51940=CARTESIAN_POINT('',(3.8075841652,2.75,-19.8100353356575));
#51941=CARTESIAN_POINT('Origin',(8.5707238638722,1.26959015522843E-8,-6.91637080940666E-8));
#51942=CARTESIAN_POINT('',(5.7631397208,2.75,-19.8100353356575));
#51943=CARTESIAN_POINT('',(4.785361943,2.75,-19.8100353356575));
#51944=CARTESIAN_POINT('',(1.,5.5,-19.2288845230294));
#51945=CARTESIAN_POINT('Origin',(10.526279440744,4.94369545300799E-10,-2.25620633287349E-9));
#51946=CARTESIAN_POINT('Origin',(-8.52627944326717,-9.62673274429449E-10,
4.51972903547926E-9));
#51947=CARTESIAN_POINT('',(-1.9747474276,-0.2016666667,-19.9989832380434));
#51948=CARTESIAN_POINT('',(-0.5561396937,2.1388888889,-19.8852999555184));
#51949=CARTESIAN_POINT('Origin',(-1.85251751839491,0.,0.));
#51950=CARTESIAN_POINT('',(-1.6994942043,2.1388888889,-19.8852999555184));
#51951=CARTESIAN_POINT('',(-1.127816949,2.1388888889,-19.8852999555184));
#51952=CARTESIAN_POINT('',(-2.785361943,0.3473197978,-19.9969839965445));
#51953=CARTESIAN_POINT('Origin',(-2.99587202900023,0.,0.));
#51954=CARTESIAN_POINT('',(-2.785361943,2.1388888889,-19.8852999555184));
#51955=CARTESIAN_POINT('Origin',(-2.785361943,0.,0.));
#51956=CARTESIAN_POINT('',(-3.7631397208,2.1388888889,-19.8852999555184));
#51957=CARTESIAN_POINT('',(-3.2742508319,2.1388888889,-19.8852999555184));
#51958=CARTESIAN_POINT('',(-3.7631397208,-2.1388888889,-19.8852999555184));
#51959=CARTESIAN_POINT('Origin',(-3.7631397208,0.,0.));
#51960=CARTESIAN_POINT('',(-2.785361943,-2.1388888889,-19.8852999555184));
#51961=CARTESIAN_POINT('',(-3.2742508319,-2.1388888889,-19.8852999555184));
#51962=CARTESIAN_POINT('',(-2.785361943,-0.7484330612,-19.9859912927256));
#51963=CARTESIAN_POINT('Origin',(-2.785361943,0.,0.));
#51964=CARTESIAN_POINT('',(-1.8474876449,-2.1388888889,-19.8852999555184));
#51965=CARTESIAN_POINT('Origin',(-3.29018641707832,0.,0.));
#51966=CARTESIAN_POINT('',(-0.6680745397,-2.1388888889,-19.8852999555184));
#51967=CARTESIAN_POINT('',(-1.2577810923,-2.1388888889,-19.8852999555184));
#51968=CARTESIAN_POINT('Origin',(-2.11077331185338,0.,0.));
#51969=CARTESIAN_POINT('',(1.,-4.3709594736,-19.5165241085637));
#51970=CARTESIAN_POINT('',(-1.8075841652,-2.75,-19.8100353356575));
#51971=CARTESIAN_POINT('Origin',(-6.57072387874695,-4.11288225699025E-9,
-2.09971195985759E-8));
#51972=CARTESIAN_POINT('',(-3.7631397208,-2.75,-19.8100353356575));
#51973=CARTESIAN_POINT('',(-2.785361943,-2.75,-19.8100353356575));
#51974=CARTESIAN_POINT('',(1.,-5.5,-19.2288845230294));
#51975=CARTESIAN_POINT('Origin',(-8.52627944334428,1.00725594531781E-9,
4.7267834091258E-9));
#51976=CARTESIAN_POINT('',(5.7631397208,-2.75,-19.8100353356575));
#51977=CARTESIAN_POINT('Origin',(10.5262794407692,-4.79505324335605E-10,
-2.19413154312065E-9));
#51978=CARTESIAN_POINT('',(3.8075841652,-2.75,-19.8100353356575));
#51979=CARTESIAN_POINT('',(4.785361943,-2.75,-19.8100353356575));
#51980=CARTESIAN_POINT('Origin',(8.57072386754017,-1.05836966968198E-8,
-5.72841307722172E-8));
#51981=CARTESIAN_POINT('Origin',(1.,0.,0.));
#51982=CARTESIAN_POINT('',(1.4888888889,2.1388888889,-19.3823413013222));
#51983=CARTESIAN_POINT('',(1.4888888889,-1.1611111111,-19.4654006120521));
#51984=CARTESIAN_POINT('Origin',(1.4888888889,0.,0.));
#51985=CARTESIAN_POINT('',(2.5277777778,-1.1611111111,-19.4654006120521));
#51986=CARTESIAN_POINT('',(2.00833333335,-1.1611111111,-19.4654006120521));
#51987=CARTESIAN_POINT('',(2.5277777778,-2.1388888889,-19.3823413013222));
#51988=CARTESIAN_POINT('Origin',(2.5277777778,0.,0.));
#51989=CARTESIAN_POINT('',(-0.5277777778,-2.1388888889,-19.3823413013222));
#51990=CARTESIAN_POINT('',(1.,-2.1388888889,-19.3823413013222));
#51991=CARTESIAN_POINT('',(-0.5277777778,-1.1611111111,-19.4654006120521));
#51992=CARTESIAN_POINT('Origin',(-0.5277777778,0.,0.));
#51993=CARTESIAN_POINT('',(0.5111111111,-1.1611111111,-19.4654006120521));
#51994=CARTESIAN_POINT('',(-0.00833333334999997,-1.1611111111,-19.4654006120521));
#51995=CARTESIAN_POINT('',(0.5111111111,2.1388888889,-19.3823413013222));
#51996=CARTESIAN_POINT('Origin',(0.5111111111,0.,0.));
#51997=CARTESIAN_POINT('',(1.,2.1388888889,-19.3823413013222));
#51998=CARTESIAN_POINT('Origin',(0.5111111111,0.4888888889,0.));
#51999=CARTESIAN_POINT('',(0.5111111111,2.1388888889,0.));
#52000=CARTESIAN_POINT('',(0.5111111111,-1.1611111111,0.));
#52001=CARTESIAN_POINT('Origin',(1.,2.1388888889,0.));
#52002=CARTESIAN_POINT('',(1.4888888889,2.1388888889,0.));
#52003=CARTESIAN_POINT('Origin',(-0.00833333334999997,-1.1611111111,0.));
#52004=CARTESIAN_POINT('',(-0.5277777778,-1.1611111111,0.));
#52005=CARTESIAN_POINT('Origin',(-0.5277777778,-1.65,0.));
#52006=CARTESIAN_POINT('',(-0.5277777778,-2.1388888889,0.));
#52007=CARTESIAN_POINT('Origin',(1.,-2.1388888889,0.));
#52008=CARTESIAN_POINT('',(2.5277777778,-2.1388888889,0.));
#52009=CARTESIAN_POINT('Origin',(2.5277777778,-1.65,0.));
#52010=CARTESIAN_POINT('',(2.5277777778,-1.1611111111,0.));
#52011=CARTESIAN_POINT('Origin',(2.00833333335,-1.1611111111,0.));
#52012=CARTESIAN_POINT('',(1.4888888889,-1.1611111111,0.));
#52013=CARTESIAN_POINT('Origin',(1.4888888889,0.4888888889,0.));
#52014=CARTESIAN_POINT('Origin',(-2.24242807365,1.24310434335,0.));
#52015=CARTESIAN_POINT('',(-1.6994942043,2.1388888889,-19.3823413013222));
#52016=CARTESIAN_POINT('',(-1.6994942043,2.1388888889,0.));
#52017=CARTESIAN_POINT('',(-2.785361943,0.3473197978,-19.4969066510064));
#52018=CARTESIAN_POINT('Origin',(-2.99587202900024,0.,0.));
#52019=CARTESIAN_POINT('',(-2.785361943,0.3473197978,0.));
#52020=CARTESIAN_POINT('Origin',(-1.127816949,2.1388888889,0.));
#52021=CARTESIAN_POINT('',(-0.5561396937,2.1388888889,-19.3823413013222));
#52022=CARTESIAN_POINT('',(-0.5561396937,2.1388888889,0.));
#52023=CARTESIAN_POINT('',(-1.127816949,2.1388888889,-19.3823413013222));
#52024=CARTESIAN_POINT('Origin',(-1.26544356065,0.9686111111,0.));
#52025=CARTESIAN_POINT('',(-1.9747474276,-0.2016666667,-19.4989571658472));
#52026=CARTESIAN_POINT('',(-1.9747474276,-0.2016666667,0.));
#52027=CARTESIAN_POINT('Origin',(-1.85251751839491,0.,0.));
#52028=CARTESIAN_POINT('Origin',(-1.2577810923,-2.1388888889,0.));
#52029=CARTESIAN_POINT('',(-1.8474876449,-2.1388888889,-19.3823413013222));
#52030=CARTESIAN_POINT('',(-1.8474876449,-2.1388888889,0.));
#52031=CARTESIAN_POINT('',(-0.6680745397,-2.1388888889,-19.3823413013222));
#52032=CARTESIAN_POINT('',(-1.2577810923,-2.1388888889,-19.3823413013222));
#52033=CARTESIAN_POINT('',(-0.6680745397,-2.1388888889,0.));
#52034=CARTESIAN_POINT('Origin',(-2.31642479395,-1.44366097505,0.));
#52035=CARTESIAN_POINT('',(-2.785361943,-0.7484330612,-19.4856318335563));
#52036=CARTESIAN_POINT('',(-2.785361943,-0.7484330612,0.));
#52037=CARTESIAN_POINT('Origin',(-3.29018641707832,0.,0.));
#52038=CARTESIAN_POINT('Origin',(-2.785361943,-1.44366097505,0.));
#52039=CARTESIAN_POINT('',(-2.785361943,-2.1388888889,-19.3823413013222));
#52040=CARTESIAN_POINT('',(-2.785361943,-2.1388888889,0.));
#52041=CARTESIAN_POINT('Origin',(-2.785361943,0.,0.));
#52042=CARTESIAN_POINT('Origin',(-3.2742508319,-2.1388888889,0.));
#52043=CARTESIAN_POINT('',(-3.7631397208,-2.1388888889,-19.3823413013222));
#52044=CARTESIAN_POINT('',(-3.7631397208,-2.1388888889,0.));
#52045=CARTESIAN_POINT('',(-3.2742508319,-2.1388888889,-19.3823413013222));
#52046=CARTESIAN_POINT('Origin',(-3.7631397208,0.,0.));
#52047=CARTESIAN_POINT('',(-3.7631397208,2.1388888889,-19.3823413013222));
#52048=CARTESIAN_POINT('',(-3.7631397208,2.1388888889,0.));
#52049=CARTESIAN_POINT('Origin',(-3.7631397208,0.,0.));
#52050=CARTESIAN_POINT('Origin',(-3.2742508319,2.1388888889,0.));
#52051=CARTESIAN_POINT('',(-2.785361943,2.1388888889,-19.3823413013222));
#52052=CARTESIAN_POINT('',(-2.785361943,2.1388888889,0.));
#52053=CARTESIAN_POINT('',(-3.2742508319,2.1388888889,-19.3823413013222));
#52054=CARTESIAN_POINT('Origin',(-2.785361943,1.24310434335,0.));
#52055=CARTESIAN_POINT('Origin',(-2.785361943,0.,0.));
#52056=CARTESIAN_POINT('Origin',(-1.32141098365,-1.1702777778,0.));
#52057=CARTESIAN_POINT('Origin',(-2.11077331185338,0.,0.));
#52058=CARTESIAN_POINT('Origin',(1.,0.,0.));
#52059=CARTESIAN_POINT('Origin',(1.,0.,0.));
#52060=CARTESIAN_POINT('',(1.,5.5,-18.7082869338697));
#52061=CARTESIAN_POINT('',(5.7631397208,2.75,-19.305115902268));
#52062=CARTESIAN_POINT('Origin',(10.5262794424987,-5.18419751571741E-10,
2.36643593609642E-9));
#52063=CARTESIAN_POINT('',(3.8075841652,2.75,-19.305115902268));
#52064=CARTESIAN_POINT('',(4.785361943,2.75,-19.305115902268));
#52065=CARTESIAN_POINT('',(1.,4.3709594736,-19.0038078626402));
#52066=CARTESIAN_POINT('Origin',(8.570723907158,-1.22962007242933E-8,6.41915343102539E-8));
#52067=CARTESIAN_POINT('',(-1.8075841652,2.75,-19.305115902268));
#52068=CARTESIAN_POINT('Origin',(-6.57072388594774,-4.93771690202038E-11,
4.65181226871891E-10));
#52069=CARTESIAN_POINT('',(-3.7631397208,2.75,-19.305115902268));
#52070=CARTESIAN_POINT('',(-2.785361943,2.75,-19.305115902268));
#52071=CARTESIAN_POINT('Origin',(-8.5262794404497,6.64190369370488E-10,
-3.11044967560292E-9));
#52072=CARTESIAN_POINT('Origin',(2.4037920826,3.5604797368,0.));
#52073=CARTESIAN_POINT('',(1.,4.3709594736,0.));
#52074=CARTESIAN_POINT('',(3.8075841652,2.75,0.));
#52075=CARTESIAN_POINT('Origin',(-0.4037920826,3.5604797368,0.));
#52076=CARTESIAN_POINT('',(-1.8075841652,2.75,0.));
#52077=CARTESIAN_POINT('Origin',(4.785361943,2.75,0.));
#52078=CARTESIAN_POINT('',(5.7631397208,2.75,0.));
#52079=CARTESIAN_POINT('Origin',(3.3815698604,4.125,0.));
#52080=CARTESIAN_POINT('',(1.,5.5,0.));
#52081=CARTESIAN_POINT('Origin',(-1.3815698604,4.125,0.));
#52082=CARTESIAN_POINT('',(-3.7631397208,2.75,0.));
#52083=CARTESIAN_POINT('Origin',(-2.785361943,2.75,0.));
#52084=CARTESIAN_POINT('Origin',(4.785361943,-2.75,0.));
#52085=CARTESIAN_POINT('',(5.7631397208,-2.75,-19.305115902268));
#52086=CARTESIAN_POINT('',(5.7631397208,-2.75,0.));
#52087=CARTESIAN_POINT('',(3.8075841652,-2.75,-19.305115902268));
#52088=CARTESIAN_POINT('',(4.785361943,-2.75,-19.305115902268));
#52089=CARTESIAN_POINT('',(3.8075841652,-2.75,0.));
#52090=CARTESIAN_POINT('Origin',(3.3815698604,-4.125,0.));
#52091=CARTESIAN_POINT('',(1.,-5.5,-18.7082869338697));
#52092=CARTESIAN_POINT('',(1.,-5.5,0.));
#52093=CARTESIAN_POINT('Origin',(10.5262794400813,-8.77110606367637E-10,
-4.09533296164E-9));
#52094=CARTESIAN_POINT('Origin',(-1.3815698604,-4.125,0.));
#52095=CARTESIAN_POINT('',(-3.7631397208,-2.75,-19.305115902268));
#52096=CARTESIAN_POINT('',(-3.7631397208,-2.75,0.));
#52097=CARTESIAN_POINT('Origin',(-8.52627944078166,-4.73031613879016E-10,
-2.23582041769532E-9));
#52098=CARTESIAN_POINT('Origin',(-2.785361943,-2.75,0.));
#52099=CARTESIAN_POINT('',(-1.8075841652,-2.75,-19.305115902268));
#52100=CARTESIAN_POINT('',(-1.8075841652,-2.75,0.));
#52101=CARTESIAN_POINT('',(-2.785361943,-2.75,-19.305115902268));
#52102=CARTESIAN_POINT('Origin',(2.4037920826,-3.5604797368,0.));
#52103=CARTESIAN_POINT('',(1.,-4.3709594736,-19.0038078626402));
#52104=CARTESIAN_POINT('Origin',(8.57072389406941,4.73950212409591E-9,2.49748000058503E-8));
#52105=CARTESIAN_POINT('',(1.,-4.3709594736,0.));
#52106=CARTESIAN_POINT('Origin',(-0.4037920826,-3.5604797368,0.));
#52107=CARTESIAN_POINT('Origin',(-6.57072389929174,7.75191022484023E-9,
4.058589020417E-8));
#52108=CARTESIAN_POINT('Origin',(1.,0.,0.));
#52109=CARTESIAN_POINT('Origin',(4.4794070911,1.4086111111,0.));
#52110=CARTESIAN_POINT('',(4.7295794663,2.1388888889,-19.3823413013222));
#52111=CARTESIAN_POINT('',(4.7295794663,2.1388888889,0.));
#52112=CARTESIAN_POINT('',(4.2292347159,0.6783333333,-19.4881980667514));
#52113=CARTESIAN_POINT('Origin',(3.99710417002144,0.000721430429313635,
2.2697089266716));
#52114=CARTESIAN_POINT('',(4.2292347159,0.6783333333,0.));
#52115=CARTESIAN_POINT('Origin',(5.24635959355,2.1388888889,0.));
#52116=CARTESIAN_POINT('',(5.7631397208,2.1388888889,-19.3823413013222));
#52117=CARTESIAN_POINT('',(5.7631397208,2.1388888889,0.));
#52118=CARTESIAN_POINT('',(5.24635959355,2.1388888889,-19.3823413013222));
#52119=CARTESIAN_POINT('Origin',(5.47540903359635,1.29897470288934,0.));
#52120=CARTESIAN_POINT('',(5.18767834635794,0.459060516890588,-19.4945957496387));
#52121=CARTESIAN_POINT('',(5.18767834635794,0.459060516890588,0.));
#52122=CARTESIAN_POINT('Origin',(5.03060343765304,0.000543454432446466,
2.27211957514992));
#52123=CARTESIAN_POINT('Origin',(4.3435534146,-0.7027777778,0.));
#52124=CARTESIAN_POINT('',(4.3435534146,-2.1388888889,-19.3823413013222));
#52125=CARTESIAN_POINT('',(4.3435534146,-2.1388888889,0.));
#52126=CARTESIAN_POINT('Ctrl Pts',(4.3435534146,-2.1388888889,-19.3823413013222));
#52127=CARTESIAN_POINT('Ctrl Pts',(4.52395809426988,-2.1388888889,-19.3823413013222));
#52128=CARTESIAN_POINT('Ctrl Pts',(4.71629563622818,-2.10281731621556,-19.3864277949426));
#52129=CARTESIAN_POINT('Ctrl Pts',(5.06994974058055,-1.95633107681449,-19.4017574464858));
#52130=CARTESIAN_POINT('Ctrl Pts',(5.23127577915034,-1.84592395078976,-19.4128536921776));
#52131=CARTESIAN_POINT('Ctrl Pts',(5.48621793448543,-1.59118019669263,-19.4353935671731));
#52132=CARTESIAN_POINT('Ctrl Pts',(5.59680474635876,-1.42973736216137,-19.4483236475342));
#52133=CARTESIAN_POINT('Ctrl Pts',(5.74353126970954,-1.07583427316188,-19.4711073706637));
#52134=CARTESIAN_POINT('Ctrl Pts',(5.7796645257,-0.883362239425408,-19.4808193953452));
#52135=CARTESIAN_POINT('Ctrl Pts',(5.7796645257,-0.522566272387348,-19.4938308937715));
#52136=CARTESIAN_POINT('Ctrl Pts',(5.74366463353765,-0.330266483099083,
-19.4980055699564));
#52137=CARTESIAN_POINT('Ctrl Pts',(5.59716211486846,0.0235426180269262,
-19.500788263579));
#52138=CARTESIAN_POINT('Ctrl Pts',(5.48665892619763,0.185050560069143,-19.4995390181328));
#52139=CARTESIAN_POINT('Ctrl Pts',(5.30716969365494,0.364587581151339,-19.4966607992451));
#52140=CARTESIAN_POINT('Ctrl Pts',(5.24968384954062,0.414010881858001,-19.495656582549));
#52141=CARTESIAN_POINT('Ctrl Pts',(5.18767834635794,0.459060516890588,-19.4945957496387));
#52142=CARTESIAN_POINT('Origin',(3.54299785905,-2.1388888889,0.));
#52143=CARTESIAN_POINT('',(2.7424423035,-2.1388888889,-19.3823413013222));
#52144=CARTESIAN_POINT('',(2.7424423035,-2.1388888889,0.));
#52145=CARTESIAN_POINT('',(3.54299785905,-2.1388888889,-19.3823413013222));
#52146=CARTESIAN_POINT('Origin',(3.7202200813,-0.7027777778,0.));
#52147=CARTESIAN_POINT('',(3.7202200813,-1.1061111111,-19.468603396492));
#52148=CARTESIAN_POINT('',(3.7202200813,-1.1061111111,0.));
#52149=CARTESIAN_POINT('',(3.7202200813,-0.2994444445,-19.497700711229));
#52150=CARTESIAN_POINT('Origin',(3.7202200813,0.,0.));
#52151=CARTESIAN_POINT('',(3.7202200813,-0.2994444445,0.));
#52152=CARTESIAN_POINT('Origin',(4.03188674795,-1.1061111111,0.));
#52153=CARTESIAN_POINT('',(4.3435534146,-1.1061111111,-19.468603396492));
#52154=CARTESIAN_POINT('',(4.3435534146,-1.1061111111,0.));
#52155=CARTESIAN_POINT('',(4.03188674795,-1.1061111111,-19.468603396492));
#52156=CARTESIAN_POINT('Origin',(2.7424423035,0.,0.));
#52157=CARTESIAN_POINT('',(2.7424423035,2.1388888889,-19.3823413013222));
#52158=CARTESIAN_POINT('',(2.7424423035,2.1388888889,0.));
#52159=CARTESIAN_POINT('Origin',(2.7424423035,0.,0.));
#52160=CARTESIAN_POINT('Origin',(3.2313311924,2.1388888889,0.));
#52161=CARTESIAN_POINT('',(3.7202200813,2.1388888889,-19.3823413013222));
#52162=CARTESIAN_POINT('',(3.7202200813,2.1388888889,0.));
#52163=CARTESIAN_POINT('',(3.2313311924,2.1388888889,-19.3823413013222));
#52164=CARTESIAN_POINT('Origin',(3.7202200813,1.4086111111,0.));
#52165=CARTESIAN_POINT('',(3.7202200813,0.6783333333,-19.4881980667514));
#52166=CARTESIAN_POINT('',(3.7202200813,0.6783333333,0.));
#52167=CARTESIAN_POINT('Origin',(3.7202200813,0.,0.));
#52168=CARTESIAN_POINT('Origin',(3.9747273986,0.6783333333,0.));
#52169=CARTESIAN_POINT('',(3.9747273986,0.6783333333,-19.4881980667514));
#52170=CARTESIAN_POINT('Origin',(4.3435534146,-0.7027777778,0.));
#52171=CARTESIAN_POINT('',(4.3435534146,-0.2994444445,-19.497700711229));
#52172=CARTESIAN_POINT('',(4.3435534146,-0.2994444445,0.));
#52173=CARTESIAN_POINT('Ctrl Pts',(4.3435534146,-1.1061111111,-19.468603396492));
#52174=CARTESIAN_POINT('Ctrl Pts',(4.39419814308983,-1.1061111111,-19.468603396492));
#52175=CARTESIAN_POINT('Ctrl Pts',(4.44821225425436,-1.0959892259289,-19.4691867368818));
#52176=CARTESIAN_POINT('Ctrl Pts',(4.54756315899303,-1.0548413233652,-19.4714594820528));
#52177=CARTESIAN_POINT('Ctrl Pts',(4.59290043242865,-1.02381583731486,-19.4731375157807));
#52178=CARTESIAN_POINT('Ctrl Pts',(4.66452631029908,-0.952218736036693,
-19.4767698957415));
#52179=CARTESIAN_POINT('Ctrl Pts',(4.69557900256288,-0.906859343552727,
-19.4789650772337));
#52180=CARTESIAN_POINT('Ctrl Pts',(4.73675930343402,-0.807469845951887,
-19.4833381841241));
#52181=CARTESIAN_POINT('Ctrl Pts',(4.7468867479,-0.75343917779947,-19.4855048515763));
#52182=CARTESIAN_POINT('Ctrl Pts',(4.7468867479,-0.652145736281435,-19.4891578288136));
#52183=CARTESIAN_POINT('Ctrl Pts',(4.73676979677675,-0.598128620436881,
-19.4908879558739));
#52184=CARTESIAN_POINT('Ctrl Pts',(4.69560712746241,-0.498746523663012,
-19.4936841838618));
#52185=CARTESIAN_POINT('Ctrl Pts',(4.66456102115108,-0.453382021110974,
-19.4947615621894));
#52186=CARTESIAN_POINT('Ctrl Pts',(4.59293064696051,-0.381759433086016,
-19.4962956016238));
#52187=CARTESIAN_POINT('Ctrl Pts',(4.54757997199792,-0.350722506379112,
-19.4968566012566));
#52188=CARTESIAN_POINT('Ctrl Pts',(4.44821221942384,-0.309565004720403,
-19.4975535161267));
#52189=CARTESIAN_POINT('Ctrl Pts',(4.39419521514208,-0.2994444445,-19.497700711229));
#52190=CARTESIAN_POINT('Ctrl Pts',(4.3435534146,-0.2994444445,-19.497700711229));
#52191=CARTESIAN_POINT('Origin',(4.03188674795,-0.2994444445,0.));
#52192=CARTESIAN_POINT('',(4.03188674795,-0.2994444445,-19.497700711229));
#52193=CARTESIAN_POINT('Origin',(1.,0.,0.));
#57022=UNCERTAINTY_MEASURE_WITH_UNIT(LENGTH_MEASURE(0.01),#57080,
'DISTANCE_ACCURACY_VALUE',
'Maximum model space distance between geometric entities at asserted c
onnectivities');
#57040=UNCERTAINTY_MEASURE_WITH_UNIT(LENGTH_MEASURE(0.01),#57080,
'DISTANCE_ACCURACY_VALUE',
'Maximum model space distance between geometric entities at asserted c
onnectivities');
#57061=(
GEOMETRIC_REPRESENTATION_CONTEXT(3)
GLOBAL_UNCERTAINTY_ASSIGNED_CONTEXT((#57022))
GLOBAL_UNIT_ASSIGNED_CONTEXT((#57080,#57082,#57083))
REPRESENTATION_CONTEXT('','3D')
);
#57079=(
GEOMETRIC_REPRESENTATION_CONTEXT(3)
GLOBAL_UNCERTAINTY_ASSIGNED_CONTEXT((#57040))
GLOBAL_UNIT_ASSIGNED_CONTEXT((#57080,#57082,#57083))
REPRESENTATION_CONTEXT('','3D')
);
#57080=(
LENGTH_UNIT()
NAMED_UNIT(*)
SI_UNIT(.MILLI.,.METRE.)
);
#57082=(
NAMED_UNIT(*)
PLANE_ANGLE_UNIT()
SI_UNIT($,.RADIAN.)
);
#57083=(
NAMED_UNIT(*)
SI_UNIT($,.STERADIAN.)
SOLID_ANGLE_UNIT()
);
#57104=SHAPE_DEFINITION_REPRESENTATION(#57150,#57269);
#57150=PRODUCT_DEFINITION_SHAPE('',$,#57308);
#57269=SHAPE_REPRESENTATION('',(#25657),#57061);
#57287=PRODUCT_DEFINITION_CONTEXT('part definition',#57403,'design');
#57308=PRODUCT_DEFINITION('Coupling Hub 1','Coupling Hub 1',#57346,#57287);
#57346=PRODUCT_DEFINITION_FORMATION('',$,#57425);
#57403=APPLICATION_CONTEXT(
'Core Data for Automotive Mechanical Design Process');
#57404=PRODUCT_CONTEXT('part definition',#57403,'mechanical');
#57425=PRODUCT('Coupling Hub 1','Coupling Hub 1',$,(#57404));
#57444=PRESENTATION_STYLE_ASSIGNMENT((#57446));
#57446=SURFACE_STYLE_USAGE(.BOTH.,#57448);
#57448=SURFACE_SIDE_STYLE('',(#57450));
#57450=SURFACE_STYLE_FILL_AREA(#57452);
#57452=FILL_AREA_STYLE('Opaque(202,209,238)',(#57454));
#57454=FILL_AREA_STYLE_COLOUR('Opaque(202,209,238)',#57456);
#57456=COLOUR_RGB('Opaque(202,209,238)',0.792156862745098,0.819607843137255,
0.933333333333333);
ENDSEC;
END-ISO-10303-21;
